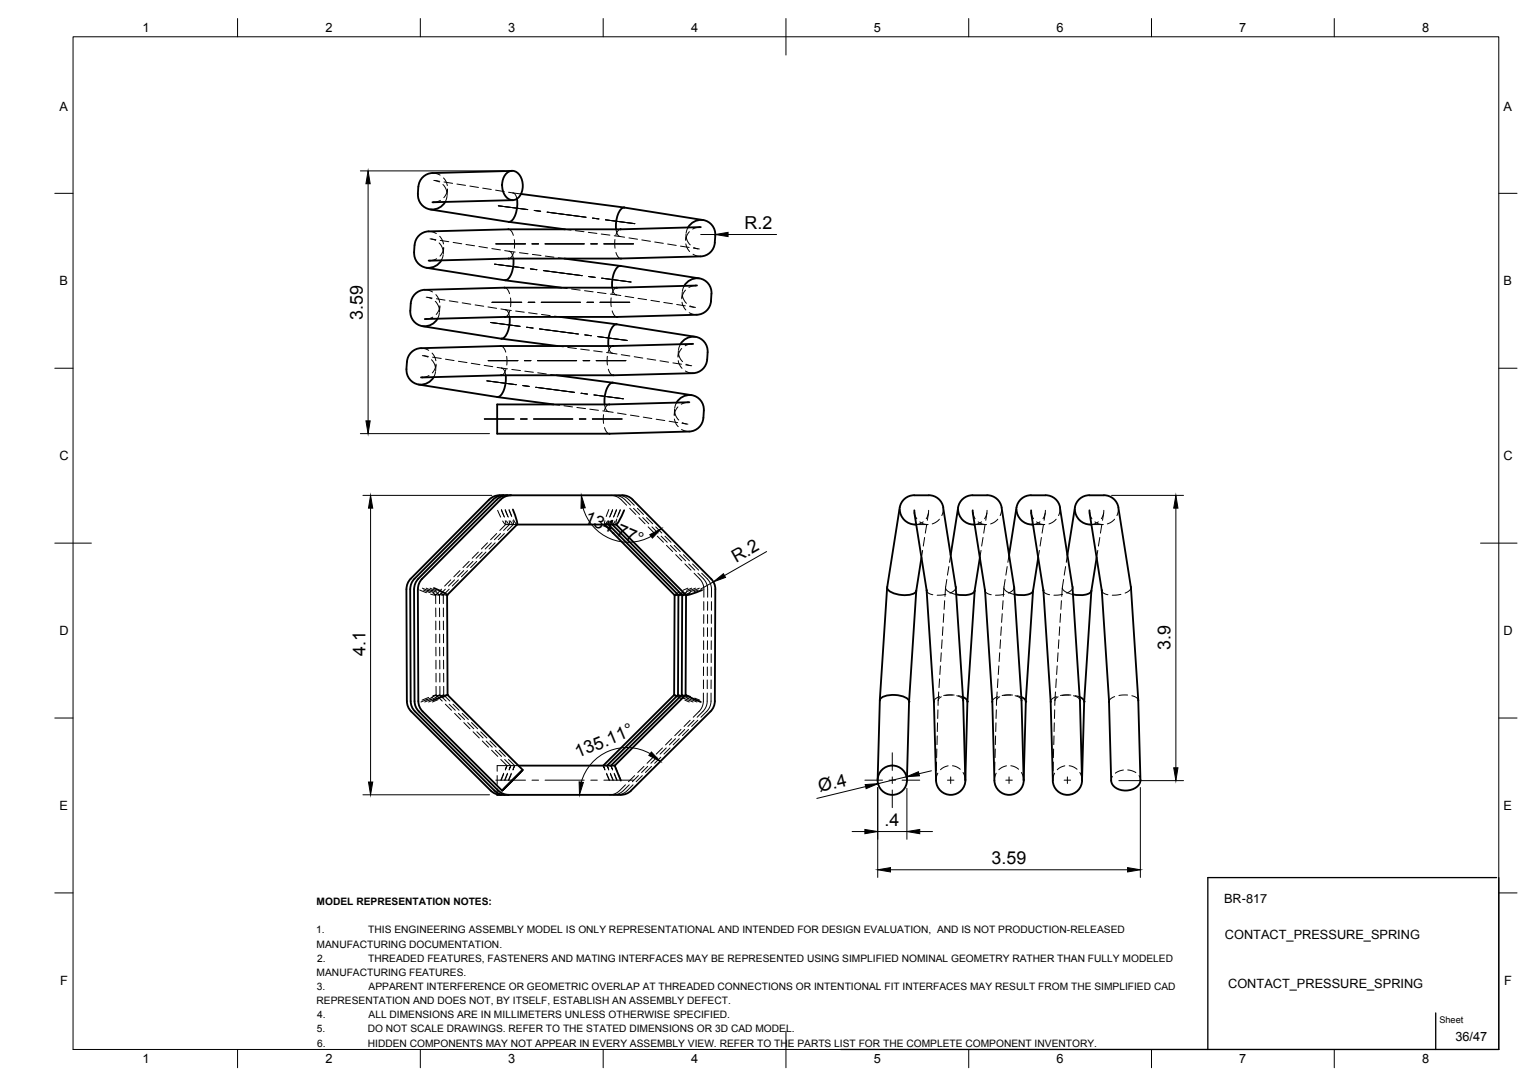
ISO-10303-21;
HEADER;
FILE_DESCRIPTION((''),'2;1');
FILE_NAME('CONTACT_PRESSURE_SPRING.step','2026-10-01T22:07:29-07:00',(''),(''),'','','');
FILE_SCHEMA (('AUTOMOTIVE_DESIGN { 1 0 10303 214 3 1 1 }'));
ENDSEC;
DATA;
#10=MECHANICAL_DESIGN_GEOMETRIC_PRESENTATION_REPRESENTATION('',(#569),#15484);
#131=ELLIPSE('',#9676,0.0216399563664951,0.02) ;
#132=ELLIPSE('',#9677,0.0216399563664951,0.02) ;
#133=ELLIPSE('',#9678,0.0216399563664951,0.02) ;
#134=ELLIPSE('',#9681,0.0216399563664949,0.02) ;
#135=ELLIPSE('',#9682,0.0216399563664949,0.02) ;
#136=ELLIPSE('',#9684,0.0216399563664949,0.02) ;
#137=ELLIPSE('',#9686,0.0216399563664949,0.02) ;
#138=ELLIPSE('',#9688,0.021639956366495,0.02) ;
#139=ELLIPSE('',#9690,0.021639956366495,0.02) ;
#140=ELLIPSE('',#9691,0.021639956366495,0.02) ;
#141=ELLIPSE('',#9693,0.0216399563664949,0.02) ;
#142=ELLIPSE('',#9694,0.0216399563664949,0.02) ;
#143=ELLIPSE('',#9695,0.0216399563664949,0.02) ;
#144=ELLIPSE('',#9697,0.021639956366495,0.02) ;
#145=ELLIPSE('',#9698,0.021639956366495,0.02) ;
#146=ELLIPSE('',#9700,0.0216399563664951,0.02) ;
#147=ELLIPSE('',#9701,0.0216399563664951,0.02) ;
#148=ELLIPSE('',#9702,0.0216399563664951,0.02) ;
#149=ELLIPSE('',#9704,0.0216399563664949,0.02) ;
#150=ELLIPSE('',#9705,0.0216399563664949,0.02) ;
#151=ELLIPSE('',#9707,0.0216399563664949,0.02) ;
#152=ELLIPSE('',#9709,0.021639956366495,0.02) ;
#153=ELLIPSE('',#9711,0.0216399563664949,0.02) ;
#154=ELLIPSE('',#9713,0.021639956366495,0.02) ;
#155=ELLIPSE('',#9714,0.021639956366495,0.02) ;
#156=ELLIPSE('',#9716,0.021639956366495,0.02) ;
#157=ELLIPSE('',#9717,0.021639956366495,0.02) ;
#158=ELLIPSE('',#9718,0.021639956366495,0.02) ;
#159=ELLIPSE('',#9720,0.021639956366495,0.02) ;
#160=ELLIPSE('',#9721,0.021639956366495,0.02) ;
#161=ELLIPSE('',#9723,0.021639956366495,0.02) ;
#162=ELLIPSE('',#9724,0.021639956366495,0.02) ;
#163=ELLIPSE('',#9725,0.021639956366495,0.02) ;
#164=ELLIPSE('',#9727,0.021639956366495,0.02) ;
#165=ELLIPSE('',#9728,0.021639956366495,0.02) ;
#166=ELLIPSE('',#9730,0.0216399563664949,0.02) ;
#167=ELLIPSE('',#9732,0.021639956366495,0.02) ;
#168=ELLIPSE('',#9734,0.0216399563664949,0.02) ;
#169=ELLIPSE('',#9736,0.021639956366495,0.02) ;
#170=ELLIPSE('',#9737,0.021639956366495,0.02) ;
#171=ELLIPSE('',#9739,0.0216399563664949,0.02) ;
#172=ELLIPSE('',#9740,0.0216399563664949,0.02) ;
#173=ELLIPSE('',#9741,0.0216399563664949,0.02) ;
#174=ELLIPSE('',#9743,0.0216399563664949,0.02) ;
#175=ELLIPSE('',#9744,0.0216399563664949,0.02) ;
#176=ELLIPSE('',#9746,0.0216399563664949,0.02) ;
#177=ELLIPSE('',#9747,0.0216399563664949,0.02) ;
#178=ELLIPSE('',#9748,0.0216399563664949,0.02) ;
#179=ELLIPSE('',#9750,0.021639956366495,0.02) ;
#180=ELLIPSE('',#9751,0.021639956366495,0.02) ;
#181=ELLIPSE('',#9753,0.0216399563664949,0.02) ;
#182=ELLIPSE('',#9755,0.0216399563664949,0.02) ;
#183=ELLIPSE('',#9757,0.0216399563664948,0.02) ;
#184=ELLIPSE('',#9759,0.021639956366495,0.02) ;
#185=ELLIPSE('',#9760,0.021639956366495,0.02) ;
#186=ELLIPSE('',#9762,0.0216399563664949,0.02) ;
#187=ELLIPSE('',#9763,0.0216399563664949,0.02) ;
#188=ELLIPSE('',#9764,0.0216399563664949,0.02) ;
#260=SPHERICAL_SURFACE('',#9549,0.02) ;
#261=SPHERICAL_SURFACE('',#9552,0.02) ;
#262=SPHERICAL_SURFACE('',#9556,0.02) ;
#263=SPHERICAL_SURFACE('',#9561,0.02) ;
#264=SPHERICAL_SURFACE('',#9566,0.02) ;
#265=SPHERICAL_SURFACE('',#9571,0.02) ;
#266=SPHERICAL_SURFACE('',#9575,0.02) ;
#267=SPHERICAL_SURFACE('',#9578,0.02) ;
#268=SPHERICAL_SURFACE('',#9581,0.02) ;
#269=SPHERICAL_SURFACE('',#9584,0.02) ;
#270=SPHERICAL_SURFACE('',#9588,0.02) ;
#271=SPHERICAL_SURFACE('',#9593,0.02) ;
#272=SPHERICAL_SURFACE('',#9598,0.02) ;
#273=SPHERICAL_SURFACE('',#9603,0.02) ;
#274=SPHERICAL_SURFACE('',#9607,0.02) ;
#275=SPHERICAL_SURFACE('',#9610,0.02) ;
#276=SPHERICAL_SURFACE('',#9613,0.02) ;
#277=SPHERICAL_SURFACE('',#9616,0.02) ;
#278=SPHERICAL_SURFACE('',#9620,0.02) ;
#279=SPHERICAL_SURFACE('',#9625,0.02) ;
#280=SPHERICAL_SURFACE('',#9630,0.02) ;
#281=SPHERICAL_SURFACE('',#9635,0.02) ;
#282=SPHERICAL_SURFACE('',#9639,0.02) ;
#283=SPHERICAL_SURFACE('',#9642,0.02) ;
#284=SPHERICAL_SURFACE('',#9645,0.02) ;
#285=SPHERICAL_SURFACE('',#9648,0.02) ;
#286=SPHERICAL_SURFACE('',#9652,0.02) ;
#287=SPHERICAL_SURFACE('',#9657,0.02) ;
#288=SPHERICAL_SURFACE('',#9662,0.02) ;
#289=SPHERICAL_SURFACE('',#9667,0.02) ;
#290=SPHERICAL_SURFACE('',#9671,0.02) ;
#498=SHAPE_REPRESENTATION_RELATIONSHIP('SRR','None',#15648,#533) ;
#533=ADVANCED_BREP_SHAPE_REPRESENTATION('',(#610),#15472) ;
#569=STYLED_ITEM('',(#15832),#610) ;
#610=MANIFOLD_SOLID_BREP('CONTACT_PRESSURE_SPRING',#8280) ;
#761=CYLINDRICAL_SURFACE('',#9674,0.02) ;
#762=CYLINDRICAL_SURFACE('',#9680,0.02) ;
#763=CYLINDRICAL_SURFACE('',#9683,0.02) ;
#764=CYLINDRICAL_SURFACE('',#9685,0.02) ;
#765=CYLINDRICAL_SURFACE('',#9687,0.02) ;
#766=CYLINDRICAL_SURFACE('',#9689,0.02) ;
#767=CYLINDRICAL_SURFACE('',#9692,0.02) ;
#768=CYLINDRICAL_SURFACE('',#9696,0.02) ;
#769=CYLINDRICAL_SURFACE('',#9699,0.02) ;
#770=CYLINDRICAL_SURFACE('',#9703,0.02) ;
#771=CYLINDRICAL_SURFACE('',#9706,0.02) ;
#772=CYLINDRICAL_SURFACE('',#9708,0.02) ;
#773=CYLINDRICAL_SURFACE('',#9710,0.02) ;
#774=CYLINDRICAL_SURFACE('',#9712,0.02) ;
#775=CYLINDRICAL_SURFACE('',#9715,0.02) ;
#776=CYLINDRICAL_SURFACE('',#9719,0.02) ;
#777=CYLINDRICAL_SURFACE('',#9722,0.02) ;
#778=CYLINDRICAL_SURFACE('',#9726,0.02) ;
#779=CYLINDRICAL_SURFACE('',#9729,0.02) ;
#780=CYLINDRICAL_SURFACE('',#9731,0.02) ;
#781=CYLINDRICAL_SURFACE('',#9733,0.02) ;
#782=CYLINDRICAL_SURFACE('',#9735,0.02) ;
#783=CYLINDRICAL_SURFACE('',#9738,0.02) ;
#784=CYLINDRICAL_SURFACE('',#9742,0.02) ;
#785=CYLINDRICAL_SURFACE('',#9745,0.02) ;
#786=CYLINDRICAL_SURFACE('',#9749,0.02) ;
#787=CYLINDRICAL_SURFACE('',#9752,0.02) ;
#788=CYLINDRICAL_SURFACE('',#9754,0.02) ;
#789=CYLINDRICAL_SURFACE('',#9756,0.02) ;
#790=CYLINDRICAL_SURFACE('',#9758,0.02) ;
#791=CYLINDRICAL_SURFACE('',#9761,0.02) ;
#792=CYLINDRICAL_SURFACE('',#9765,0.02) ;
#1229=CIRCLE('',#9550,0.02) ;
#1230=CIRCLE('',#9551,0.02) ;
#1231=CIRCLE('',#9553,0.02) ;
#1232=CIRCLE('',#9554,0.02) ;
#1233=CIRCLE('',#9555,0.02) ;
#1234=CIRCLE('',#9557,0.02) ;
#1235=CIRCLE('',#9558,0.02) ;
#1236=CIRCLE('',#9559,0.02) ;
#1237=CIRCLE('',#9560,0.02) ;
#1238=CIRCLE('',#9562,0.02) ;
#1239=CIRCLE('',#9563,0.02) ;
#1240=CIRCLE('',#9564,0.02) ;
#1241=CIRCLE('',#9565,0.02) ;
#1242=CIRCLE('',#9567,0.02) ;
#1243=CIRCLE('',#9568,0.02) ;
#1244=CIRCLE('',#9569,0.02) ;
#1245=CIRCLE('',#9570,0.02) ;
#1246=CIRCLE('',#9572,0.02) ;
#1247=CIRCLE('',#9573,0.02) ;
#1248=CIRCLE('',#9574,0.02) ;
#1249=CIRCLE('',#9576,0.02) ;
#1250=CIRCLE('',#9577,0.02) ;
#1251=CIRCLE('',#9579,0.02) ;
#1252=CIRCLE('',#9580,0.02) ;
#1253=CIRCLE('',#9582,0.02) ;
#1254=CIRCLE('',#9583,0.02) ;
#1255=CIRCLE('',#9585,0.02) ;
#1256=CIRCLE('',#9586,0.02) ;
#1257=CIRCLE('',#9587,0.02) ;
#1258=CIRCLE('',#9589,0.02) ;
#1259=CIRCLE('',#9590,0.02) ;
#1260=CIRCLE('',#9591,0.02) ;
#1261=CIRCLE('',#9592,0.02) ;
#1262=CIRCLE('',#9594,0.02) ;
#1263=CIRCLE('',#9595,0.02) ;
#1264=CIRCLE('',#9596,0.02) ;
#1265=CIRCLE('',#9597,0.02) ;
#1266=CIRCLE('',#9599,0.02) ;
#1267=CIRCLE('',#9600,0.02) ;
#1268=CIRCLE('',#9601,0.02) ;
#1269=CIRCLE('',#9602,0.02) ;
#1270=CIRCLE('',#9604,0.02) ;
#1271=CIRCLE('',#9605,0.02) ;
#1272=CIRCLE('',#9606,0.02) ;
#1273=CIRCLE('',#9608,0.02) ;
#1274=CIRCLE('',#9609,0.02) ;
#1275=CIRCLE('',#9611,0.02) ;
#1276=CIRCLE('',#9612,0.02) ;
#1277=CIRCLE('',#9614,0.02) ;
#1278=CIRCLE('',#9615,0.02) ;
#1279=CIRCLE('',#9617,0.02) ;
#1280=CIRCLE('',#9618,0.02) ;
#1281=CIRCLE('',#9619,0.02) ;
#1282=CIRCLE('',#9621,0.02) ;
#1283=CIRCLE('',#9622,0.02) ;
#1284=CIRCLE('',#9623,0.02) ;
#1285=CIRCLE('',#9624,0.02) ;
#1286=CIRCLE('',#9626,0.02) ;
#1287=CIRCLE('',#9627,0.02) ;
#1288=CIRCLE('',#9628,0.02) ;
#1289=CIRCLE('',#9629,0.02) ;
#1290=CIRCLE('',#9631,0.02) ;
#1291=CIRCLE('',#9632,0.02) ;
#1292=CIRCLE('',#9633,0.02) ;
#1293=CIRCLE('',#9634,0.02) ;
#1294=CIRCLE('',#9636,0.02) ;
#1295=CIRCLE('',#9637,0.02) ;
#1296=CIRCLE('',#9638,0.02) ;
#1297=CIRCLE('',#9640,0.02) ;
#1298=CIRCLE('',#9641,0.02) ;
#1299=CIRCLE('',#9643,0.02) ;
#1300=CIRCLE('',#9644,0.02) ;
#1301=CIRCLE('',#9646,0.02) ;
#1302=CIRCLE('',#9647,0.02) ;
#1303=CIRCLE('',#9649,0.02) ;
#1304=CIRCLE('',#9650,0.02) ;
#1305=CIRCLE('',#9651,0.02) ;
#1306=CIRCLE('',#9653,0.02) ;
#1307=CIRCLE('',#9654,0.02) ;
#1308=CIRCLE('',#9655,0.02) ;
#1309=CIRCLE('',#9656,0.02) ;
#1310=CIRCLE('',#9658,0.02) ;
#1311=CIRCLE('',#9659,0.02) ;
#1312=CIRCLE('',#9660,0.02) ;
#1313=CIRCLE('',#9661,0.02) ;
#1314=CIRCLE('',#9663,0.02) ;
#1315=CIRCLE('',#9664,0.02) ;
#1316=CIRCLE('',#9665,0.02) ;
#1317=CIRCLE('',#9666,0.02) ;
#1318=CIRCLE('',#9668,0.02) ;
#1319=CIRCLE('',#9669,0.02) ;
#1320=CIRCLE('',#9670,0.02) ;
#1321=CIRCLE('',#9672,0.02) ;
#1322=CIRCLE('',#9673,0.02) ;
#1323=CIRCLE('',#9675,0.02) ;
#1324=CIRCLE('',#9766,0.02) ;
#1724=FACE_OUTER_BOUND('',#2290,.T.) ;
#1725=FACE_OUTER_BOUND('',#2291,.T.) ;
#1726=FACE_OUTER_BOUND('',#2292,.T.) ;
#1727=FACE_OUTER_BOUND('',#2293,.T.) ;
#1728=FACE_OUTER_BOUND('',#2294,.T.) ;
#1729=FACE_OUTER_BOUND('',#2295,.T.) ;
#1730=FACE_OUTER_BOUND('',#2296,.T.) ;
#1731=FACE_OUTER_BOUND('',#2297,.T.) ;
#1732=FACE_OUTER_BOUND('',#2298,.T.) ;
#1733=FACE_OUTER_BOUND('',#2299,.T.) ;
#1734=FACE_OUTER_BOUND('',#2300,.T.) ;
#1735=FACE_OUTER_BOUND('',#2301,.T.) ;
#1736=FACE_OUTER_BOUND('',#2302,.T.) ;
#1737=FACE_OUTER_BOUND('',#2303,.T.) ;
#1738=FACE_OUTER_BOUND('',#2304,.T.) ;
#1739=FACE_OUTER_BOUND('',#2305,.T.) ;
#1740=FACE_OUTER_BOUND('',#2306,.T.) ;
#1741=FACE_OUTER_BOUND('',#2307,.T.) ;
#1742=FACE_OUTER_BOUND('',#2308,.T.) ;
#1743=FACE_OUTER_BOUND('',#2309,.T.) ;
#1744=FACE_OUTER_BOUND('',#2310,.T.) ;
#1745=FACE_OUTER_BOUND('',#2311,.T.) ;
#1746=FACE_OUTER_BOUND('',#2312,.T.) ;
#1747=FACE_OUTER_BOUND('',#2313,.T.) ;
#1748=FACE_OUTER_BOUND('',#2314,.T.) ;
#1749=FACE_OUTER_BOUND('',#2315,.T.) ;
#1750=FACE_OUTER_BOUND('',#2316,.T.) ;
#1751=FACE_OUTER_BOUND('',#2317,.T.) ;
#1752=FACE_OUTER_BOUND('',#2318,.T.) ;
#1753=FACE_OUTER_BOUND('',#2319,.T.) ;
#1754=FACE_OUTER_BOUND('',#2320,.T.) ;
#1755=FACE_OUTER_BOUND('',#2321,.T.) ;
#1756=FACE_OUTER_BOUND('',#2322,.T.) ;
#1757=FACE_OUTER_BOUND('',#2323,.T.) ;
#1758=FACE_OUTER_BOUND('',#2324,.T.) ;
#1759=FACE_OUTER_BOUND('',#2325,.T.) ;
#1760=FACE_OUTER_BOUND('',#2326,.T.) ;
#1761=FACE_OUTER_BOUND('',#2327,.T.) ;
#1762=FACE_OUTER_BOUND('',#2328,.T.) ;
#1763=FACE_OUTER_BOUND('',#2329,.T.) ;
#1764=FACE_OUTER_BOUND('',#2330,.T.) ;
#1765=FACE_OUTER_BOUND('',#2331,.T.) ;
#1766=FACE_OUTER_BOUND('',#2332,.T.) ;
#1767=FACE_OUTER_BOUND('',#2333,.T.) ;
#1768=FACE_OUTER_BOUND('',#2334,.T.) ;
#1769=FACE_OUTER_BOUND('',#2335,.T.) ;
#1770=FACE_OUTER_BOUND('',#2336,.T.) ;
#1771=FACE_OUTER_BOUND('',#2337,.T.) ;
#1772=FACE_OUTER_BOUND('',#2338,.T.) ;
#1773=FACE_OUTER_BOUND('',#2339,.T.) ;
#1774=FACE_OUTER_BOUND('',#2340,.T.) ;
#1775=FACE_OUTER_BOUND('',#2341,.T.) ;
#1776=FACE_OUTER_BOUND('',#2342,.T.) ;
#1777=FACE_OUTER_BOUND('',#2343,.T.) ;
#1778=FACE_OUTER_BOUND('',#2344,.T.) ;
#1779=FACE_OUTER_BOUND('',#2345,.T.) ;
#1780=FACE_OUTER_BOUND('',#2346,.T.) ;
#1781=FACE_OUTER_BOUND('',#2347,.T.) ;
#1782=FACE_OUTER_BOUND('',#2348,.T.) ;
#1783=FACE_OUTER_BOUND('',#2349,.T.) ;
#1784=FACE_OUTER_BOUND('',#2350,.T.) ;
#1785=FACE_OUTER_BOUND('',#2351,.T.) ;
#1786=FACE_OUTER_BOUND('',#2352,.T.) ;
#1787=FACE_OUTER_BOUND('',#2353,.T.) ;
#1788=FACE_OUTER_BOUND('',#2354,.T.) ;
#2290=EDGE_LOOP('',(#6897,#6898)) ;
#2291=EDGE_LOOP('',(#6899,#6900,#6901)) ;
#2292=EDGE_LOOP('',(#6902,#6903,#6904,#6905)) ;
#2293=EDGE_LOOP('',(#6906,#6907,#6908,#6909)) ;
#2294=EDGE_LOOP('',(#6910,#6911,#6912,#6913)) ;
#2295=EDGE_LOOP('',(#6914,#6915,#6916)) ;
#2296=EDGE_LOOP('',(#6917,#6918)) ;
#2297=EDGE_LOOP('',(#6919,#6920)) ;
#2298=EDGE_LOOP('',(#6921,#6922)) ;
#2299=EDGE_LOOP('',(#6923,#6924,#6925)) ;
#2300=EDGE_LOOP('',(#6926,#6927,#6928,#6929)) ;
#2301=EDGE_LOOP('',(#6930,#6931,#6932,#6933)) ;
#2302=EDGE_LOOP('',(#6934,#6935,#6936,#6937)) ;
#2303=EDGE_LOOP('',(#6938,#6939,#6940)) ;
#2304=EDGE_LOOP('',(#6941,#6942)) ;
#2305=EDGE_LOOP('',(#6943,#6944)) ;
#2306=EDGE_LOOP('',(#6945,#6946)) ;
#2307=EDGE_LOOP('',(#6947,#6948,#6949)) ;
#2308=EDGE_LOOP('',(#6950,#6951,#6952,#6953)) ;
#2309=EDGE_LOOP('',(#6954,#6955,#6956,#6957)) ;
#2310=EDGE_LOOP('',(#6958,#6959,#6960,#6961)) ;
#2311=EDGE_LOOP('',(#6962,#6963,#6964)) ;
#2312=EDGE_LOOP('',(#6965,#6966)) ;
#2313=EDGE_LOOP('',(#6967,#6968)) ;
#2314=EDGE_LOOP('',(#6969,#6970)) ;
#2315=EDGE_LOOP('',(#6971,#6972,#6973)) ;
#2316=EDGE_LOOP('',(#6974,#6975,#6976,#6977)) ;
#2317=EDGE_LOOP('',(#6978,#6979,#6980,#6981)) ;
#2318=EDGE_LOOP('',(#6982,#6983,#6984,#6985)) ;
#2319=EDGE_LOOP('',(#6986,#6987,#6988)) ;
#2320=EDGE_LOOP('',(#6989,#6990)) ;
#2321=EDGE_LOOP('',(#6991,#6992,#6993,#6994,#6995,#6996,#6997)) ;
#2322=EDGE_LOOP('',(#6998)) ;
#2323=EDGE_LOOP('',(#6999,#7000,#7001,#7002,#7003,#7004,#7005,#7006,#7007)) ;
#2324=EDGE_LOOP('',(#7008,#7009,#7010,#7011,#7012,#7013,#7014,#7015,#7016)) ;
#2325=EDGE_LOOP('',(#7017,#7018,#7019,#7020,#7021,#7022,#7023,#7024)) ;
#2326=EDGE_LOOP('',(#7025,#7026,#7027,#7028,#7029,#7030,#7031,#7032)) ;
#2327=EDGE_LOOP('',(#7033,#7034,#7035,#7036,#7037,#7038,#7039,#7040,#7041)) ;
#2328=EDGE_LOOP('',(#7042,#7043,#7044,#7045,#7046,#7047,#7048,#7049,#7050)) ;
#2329=EDGE_LOOP('',(#7051,#7052,#7053,#7054,#7055,#7056,#7057,#7058,#7059)) ;
#2330=EDGE_LOOP('',(#7060,#7061,#7062,#7063,#7064,#7065,#7066,#7067,#7068)) ;
#2331=EDGE_LOOP('',(#7069,#7070,#7071,#7072,#7073,#7074,#7075,#7076,#7077)) ;
#2332=EDGE_LOOP('',(#7078,#7079,#7080,#7081,#7082,#7083,#7084,#7085,#7086)) ;
#2333=EDGE_LOOP('',(#7087,#7088,#7089,#7090,#7091,#7092,#7093,#7094)) ;
#2334=EDGE_LOOP('',(#7095,#7096,#7097,#7098,#7099,#7100,#7101,#7102)) ;
#2335=EDGE_LOOP('',(#7103,#7104,#7105,#7106,#7107,#7108,#7109,#7110,#7111)) ;
#2336=EDGE_LOOP('',(#7112,#7113,#7114,#7115,#7116,#7117,#7118,#7119,#7120)) ;
#2337=EDGE_LOOP('',(#7121,#7122,#7123,#7124,#7125,#7126,#7127,#7128,#7129)) ;
#2338=EDGE_LOOP('',(#7130,#7131,#7132,#7133,#7134,#7135,#7136,#7137,#7138)) ;
#2339=EDGE_LOOP('',(#7139,#7140,#7141,#7142,#7143,#7144,#7145,#7146,#7147)) ;
#2340=EDGE_LOOP('',(#7148,#7149,#7150,#7151,#7152,#7153,#7154,#7155,#7156)) ;
#2341=EDGE_LOOP('',(#7157,#7158,#7159,#7160,#7161,#7162,#7163,#7164)) ;
#2342=EDGE_LOOP('',(#7165,#7166,#7167,#7168,#7169,#7170,#7171,#7172)) ;
#2343=EDGE_LOOP('',(#7173,#7174,#7175,#7176,#7177,#7178,#7179,#7180,#7181)) ;
#2344=EDGE_LOOP('',(#7182,#7183,#7184,#7185,#7186,#7187,#7188,#7189,#7190)) ;
#2345=EDGE_LOOP('',(#7191,#7192,#7193,#7194,#7195,#7196,#7197,#7198,#7199)) ;
#2346=EDGE_LOOP('',(#7200,#7201,#7202,#7203,#7204,#7205,#7206,#7207,#7208)) ;
#2347=EDGE_LOOP('',(#7209,#7210,#7211,#7212,#7213,#7214,#7215,#7216,#7217)) ;
#2348=EDGE_LOOP('',(#7218,#7219,#7220,#7221,#7222,#7223,#7224,#7225,#7226)) ;
#2349=EDGE_LOOP('',(#7227,#7228,#7229,#7230,#7231,#7232,#7233,#7234)) ;
#2350=EDGE_LOOP('',(#7235,#7236,#7237,#7238,#7239,#7240,#7241,#7242)) ;
#2351=EDGE_LOOP('',(#7243,#7244,#7245,#7246,#7247,#7248,#7249,#7250,#7251)) ;
#2352=EDGE_LOOP('',(#7252,#7253,#7254,#7255,#7256,#7257,#7258,#7259,#7260)) ;
#2353=EDGE_LOOP('',(#7261,#7262,#7263,#7264,#7265,#7266,#7267)) ;
#2354=EDGE_LOOP('',(#7268)) ;
#2788=LINE('',#14908,#3262) ;
#2789=LINE('',#14916,#3263) ;
#2790=LINE('',#14920,#3264) ;
#2791=LINE('',#14923,#3265) ;
#2792=LINE('',#14926,#3266) ;
#2793=LINE('',#14929,#3267) ;
#2794=LINE('',#14935,#3268) ;
#2795=LINE('',#14942,#3269) ;
#2796=LINE('',#14947,#3270) ;
#2797=LINE('',#14954,#3271) ;
#2798=LINE('',#14958,#3272) ;
#2799=LINE('',#14961,#3273) ;
#2800=LINE('',#14964,#3274) ;
#2801=LINE('',#14967,#3275) ;
#2802=LINE('',#14973,#3276) ;
#2803=LINE('',#14980,#3277) ;
#2804=LINE('',#14985,#3278) ;
#2805=LINE('',#14992,#3279) ;
#2806=LINE('',#14996,#3280) ;
#2807=LINE('',#14999,#3281) ;
#2808=LINE('',#15002,#3282) ;
#2809=LINE('',#15005,#3283) ;
#2810=LINE('',#15011,#3284) ;
#2811=LINE('',#15018,#3285) ;
#2812=LINE('',#15023,#3286) ;
#2813=LINE('',#15030,#3287) ;
#2814=LINE('',#15034,#3288) ;
#2815=LINE('',#15037,#3289) ;
#2816=LINE('',#15040,#3290) ;
#2817=LINE('',#15043,#3291) ;
#2818=LINE('',#15049,#3292) ;
#2819=LINE('',#15056,#3293) ;
#3262=VECTOR('',#12261,0.02) ;
#3263=VECTOR('',#12272,0.02) ;
#3264=VECTOR('',#12279,0.02) ;
#3265=VECTOR('',#12284,0.02) ;
#3266=VECTOR('',#12289,0.02) ;
#3267=VECTOR('',#12294,0.02) ;
#3268=VECTOR('',#12301,0.02) ;
#3269=VECTOR('',#12310,0.02) ;
#3270=VECTOR('',#12317,0.02) ;
#3271=VECTOR('',#12326,0.02) ;
#3272=VECTOR('',#12333,0.02) ;
#3273=VECTOR('',#12338,0.02) ;
#3274=VECTOR('',#12343,0.02) ;
#3275=VECTOR('',#12348,0.02) ;
#3276=VECTOR('',#12355,0.02) ;
#3277=VECTOR('',#12364,0.02) ;
#3278=VECTOR('',#12371,0.02) ;
#3279=VECTOR('',#12380,0.02) ;
#3280=VECTOR('',#12387,0.02) ;
#3281=VECTOR('',#12392,0.02) ;
#3282=VECTOR('',#12397,0.02) ;
#3283=VECTOR('',#12402,0.02) ;
#3284=VECTOR('',#12409,0.02) ;
#3285=VECTOR('',#12418,0.02) ;
#3286=VECTOR('',#12425,0.02) ;
#3287=VECTOR('',#12434,0.02) ;
#3288=VECTOR('',#12441,0.02) ;
#3289=VECTOR('',#12446,0.02) ;
#3290=VECTOR('',#12451,0.02) ;
#3291=VECTOR('',#12456,0.02) ;
#3292=VECTOR('',#12463,0.02) ;
#3293=VECTOR('',#12472,0.02) ;
#3929=VERTEX_POINT('',#14686) ;
#3930=VERTEX_POINT('',#14687) ;
#3931=VERTEX_POINT('',#14691) ;
#3932=VERTEX_POINT('',#14692) ;
#3933=VERTEX_POINT('',#14694) ;
#3934=VERTEX_POINT('',#14698) ;
#3935=VERTEX_POINT('',#14699) ;
#3936=VERTEX_POINT('',#14701) ;
#3937=VERTEX_POINT('',#14703) ;
#3938=VERTEX_POINT('',#14707) ;
#3939=VERTEX_POINT('',#14708) ;
#3940=VERTEX_POINT('',#14710) ;
#3941=VERTEX_POINT('',#14712) ;
#3942=VERTEX_POINT('',#14716) ;
#3943=VERTEX_POINT('',#14717) ;
#3944=VERTEX_POINT('',#14719) ;
#3945=VERTEX_POINT('',#14721) ;
#3946=VERTEX_POINT('',#14725) ;
#3947=VERTEX_POINT('',#14726) ;
#3948=VERTEX_POINT('',#14728) ;
#3949=VERTEX_POINT('',#14732) ;
#3950=VERTEX_POINT('',#14733) ;
#3951=VERTEX_POINT('',#14737) ;
#3952=VERTEX_POINT('',#14738) ;
#3953=VERTEX_POINT('',#14742) ;
#3954=VERTEX_POINT('',#14743) ;
#3955=VERTEX_POINT('',#14747) ;
#3956=VERTEX_POINT('',#14748) ;
#3957=VERTEX_POINT('',#14750) ;
#3958=VERTEX_POINT('',#14754) ;
#3959=VERTEX_POINT('',#14755) ;
#3960=VERTEX_POINT('',#14757) ;
#3961=VERTEX_POINT('',#14759) ;
#3962=VERTEX_POINT('',#14763) ;
#3963=VERTEX_POINT('',#14764) ;
#3964=VERTEX_POINT('',#14766) ;
#3965=VERTEX_POINT('',#14768) ;
#3966=VERTEX_POINT('',#14772) ;
#3967=VERTEX_POINT('',#14773) ;
#3968=VERTEX_POINT('',#14775) ;
#3969=VERTEX_POINT('',#14777) ;
#3970=VERTEX_POINT('',#14781) ;
#3971=VERTEX_POINT('',#14782) ;
#3972=VERTEX_POINT('',#14784) ;
#3973=VERTEX_POINT('',#14788) ;
#3974=VERTEX_POINT('',#14789) ;
#3975=VERTEX_POINT('',#14793) ;
#3976=VERTEX_POINT('',#14794) ;
#3977=VERTEX_POINT('',#14798) ;
#3978=VERTEX_POINT('',#14799) ;
#3979=VERTEX_POINT('',#14803) ;
#3980=VERTEX_POINT('',#14804) ;
#3981=VERTEX_POINT('',#14806) ;
#3982=VERTEX_POINT('',#14810) ;
#3983=VERTEX_POINT('',#14811) ;
#3984=VERTEX_POINT('',#14813) ;
#3985=VERTEX_POINT('',#14815) ;
#3986=VERTEX_POINT('',#14819) ;
#3987=VERTEX_POINT('',#14820) ;
#3988=VERTEX_POINT('',#14822) ;
#3989=VERTEX_POINT('',#14824) ;
#3990=VERTEX_POINT('',#14828) ;
#3991=VERTEX_POINT('',#14829) ;
#3992=VERTEX_POINT('',#14831) ;
#3993=VERTEX_POINT('',#14833) ;
#3994=VERTEX_POINT('',#14837) ;
#3995=VERTEX_POINT('',#14838) ;
#3996=VERTEX_POINT('',#14840) ;
#3997=VERTEX_POINT('',#14844) ;
#3998=VERTEX_POINT('',#14845) ;
#3999=VERTEX_POINT('',#14849) ;
#4000=VERTEX_POINT('',#14850) ;
#4001=VERTEX_POINT('',#14854) ;
#4002=VERTEX_POINT('',#14855) ;
#4003=VERTEX_POINT('',#14859) ;
#4004=VERTEX_POINT('',#14860) ;
#4005=VERTEX_POINT('',#14862) ;
#4006=VERTEX_POINT('',#14866) ;
#4007=VERTEX_POINT('',#14867) ;
#4008=VERTEX_POINT('',#14869) ;
#4009=VERTEX_POINT('',#14871) ;
#4010=VERTEX_POINT('',#14875) ;
#4011=VERTEX_POINT('',#14876) ;
#4012=VERTEX_POINT('',#14878) ;
#4013=VERTEX_POINT('',#14880) ;
#4014=VERTEX_POINT('',#14884) ;
#4015=VERTEX_POINT('',#14885) ;
#4016=VERTEX_POINT('',#14887) ;
#4017=VERTEX_POINT('',#14889) ;
#4018=VERTEX_POINT('',#14893) ;
#4019=VERTEX_POINT('',#14894) ;
#4020=VERTEX_POINT('',#14896) ;
#4021=VERTEX_POINT('',#14900) ;
#4022=VERTEX_POINT('',#14901) ;
#4023=VERTEX_POINT('',#14905) ;
#4024=VERTEX_POINT('',#14907) ;
#4025=VERTEX_POINT('',#14909) ;
#4026=VERTEX_POINT('',#14915) ;
#4027=VERTEX_POINT('',#14930) ;
#4028=VERTEX_POINT('',#14934) ;
#4029=VERTEX_POINT('',#14936) ;
#4030=VERTEX_POINT('',#14941) ;
#4031=VERTEX_POINT('',#14946) ;
#4032=VERTEX_POINT('',#14948) ;
#4033=VERTEX_POINT('',#14953) ;
#4034=VERTEX_POINT('',#14968) ;
#4035=VERTEX_POINT('',#14972) ;
#4036=VERTEX_POINT('',#14974) ;
#4037=VERTEX_POINT('',#14979) ;
#4038=VERTEX_POINT('',#14984) ;
#4039=VERTEX_POINT('',#14986) ;
#4040=VERTEX_POINT('',#14991) ;
#4041=VERTEX_POINT('',#15006) ;
#4042=VERTEX_POINT('',#15010) ;
#4043=VERTEX_POINT('',#15012) ;
#4044=VERTEX_POINT('',#15017) ;
#4045=VERTEX_POINT('',#15022) ;
#4046=VERTEX_POINT('',#15024) ;
#4047=VERTEX_POINT('',#15029) ;
#4048=VERTEX_POINT('',#15044) ;
#4049=VERTEX_POINT('',#15048) ;
#4050=VERTEX_POINT('',#15050) ;
#4051=VERTEX_POINT('',#15055) ;
#4953=EDGE_CURVE('',#3929,#3930,#1229,.T.) ;
#4954=EDGE_CURVE('',#3930,#3929,#1230,.T.) ;
#4955=EDGE_CURVE('',#3931,#3932,#1231,.T.) ;
#4956=EDGE_CURVE('',#3932,#3933,#1232,.T.) ;
#4957=EDGE_CURVE('',#3933,#3931,#1233,.T.) ;
#4958=EDGE_CURVE('',#3934,#3935,#1234,.T.) ;
#4959=EDGE_CURVE('',#3935,#3936,#1235,.T.) ;
#4960=EDGE_CURVE('',#3936,#3937,#1236,.T.) ;
#4961=EDGE_CURVE('',#3937,#3934,#1237,.T.) ;
#4962=EDGE_CURVE('',#3938,#3939,#1238,.T.) ;
#4963=EDGE_CURVE('',#3939,#3940,#1239,.T.) ;
#4964=EDGE_CURVE('',#3940,#3941,#1240,.T.) ;
#4965=EDGE_CURVE('',#3941,#3938,#1241,.T.) ;
#4966=EDGE_CURVE('',#3942,#3943,#1242,.T.) ;
#4967=EDGE_CURVE('',#3943,#3944,#1243,.T.) ;
#4968=EDGE_CURVE('',#3944,#3945,#1244,.T.) ;
#4969=EDGE_CURVE('',#3945,#3942,#1245,.T.) ;
#4970=EDGE_CURVE('',#3946,#3947,#1246,.T.) ;
#4971=EDGE_CURVE('',#3947,#3948,#1247,.T.) ;
#4972=EDGE_CURVE('',#3948,#3946,#1248,.T.) ;
#4973=EDGE_CURVE('',#3949,#3950,#1249,.T.) ;
#4974=EDGE_CURVE('',#3950,#3949,#1250,.T.) ;
#4975=EDGE_CURVE('',#3951,#3952,#1251,.T.) ;
#4976=EDGE_CURVE('',#3952,#3951,#1252,.T.) ;
#4977=EDGE_CURVE('',#3953,#3954,#1253,.T.) ;
#4978=EDGE_CURVE('',#3954,#3953,#1254,.T.) ;
#4979=EDGE_CURVE('',#3955,#3956,#1255,.T.) ;
#4980=EDGE_CURVE('',#3956,#3957,#1256,.T.) ;
#4981=EDGE_CURVE('',#3957,#3955,#1257,.T.) ;
#4982=EDGE_CURVE('',#3958,#3959,#1258,.T.) ;
#4983=EDGE_CURVE('',#3959,#3960,#1259,.T.) ;
#4984=EDGE_CURVE('',#3960,#3961,#1260,.T.) ;
#4985=EDGE_CURVE('',#3961,#3958,#1261,.T.) ;
#4986=EDGE_CURVE('',#3962,#3963,#1262,.T.) ;
#4987=EDGE_CURVE('',#3963,#3964,#1263,.T.) ;
#4988=EDGE_CURVE('',#3964,#3965,#1264,.T.) ;
#4989=EDGE_CURVE('',#3965,#3962,#1265,.T.) ;
#4990=EDGE_CURVE('',#3966,#3967,#1266,.T.) ;
#4991=EDGE_CURVE('',#3967,#3968,#1267,.T.) ;
#4992=EDGE_CURVE('',#3968,#3969,#1268,.T.) ;
#4993=EDGE_CURVE('',#3969,#3966,#1269,.T.) ;
#4994=EDGE_CURVE('',#3970,#3971,#1270,.T.) ;
#4995=EDGE_CURVE('',#3971,#3972,#1271,.T.) ;
#4996=EDGE_CURVE('',#3972,#3970,#1272,.T.) ;
#4997=EDGE_CURVE('',#3973,#3974,#1273,.T.) ;
#4998=EDGE_CURVE('',#3974,#3973,#1274,.T.) ;
#4999=EDGE_CURVE('',#3975,#3976,#1275,.T.) ;
#5000=EDGE_CURVE('',#3976,#3975,#1276,.T.) ;
#5001=EDGE_CURVE('',#3977,#3978,#1277,.T.) ;
#5002=EDGE_CURVE('',#3978,#3977,#1278,.T.) ;
#5003=EDGE_CURVE('',#3979,#3980,#1279,.T.) ;
#5004=EDGE_CURVE('',#3980,#3981,#1280,.T.) ;
#5005=EDGE_CURVE('',#3981,#3979,#1281,.T.) ;
#5006=EDGE_CURVE('',#3982,#3983,#1282,.T.) ;
#5007=EDGE_CURVE('',#3983,#3984,#1283,.T.) ;
#5008=EDGE_CURVE('',#3984,#3985,#1284,.T.) ;
#5009=EDGE_CURVE('',#3985,#3982,#1285,.T.) ;
#5010=EDGE_CURVE('',#3986,#3987,#1286,.T.) ;
#5011=EDGE_CURVE('',#3987,#3988,#1287,.T.) ;
#5012=EDGE_CURVE('',#3988,#3989,#1288,.T.) ;
#5013=EDGE_CURVE('',#3989,#3986,#1289,.T.) ;
#5014=EDGE_CURVE('',#3990,#3991,#1290,.T.) ;
#5015=EDGE_CURVE('',#3991,#3992,#1291,.T.) ;
#5016=EDGE_CURVE('',#3992,#3993,#1292,.T.) ;
#5017=EDGE_CURVE('',#3993,#3990,#1293,.T.) ;
#5018=EDGE_CURVE('',#3994,#3995,#1294,.T.) ;
#5019=EDGE_CURVE('',#3995,#3996,#1295,.T.) ;
#5020=EDGE_CURVE('',#3996,#3994,#1296,.T.) ;
#5021=EDGE_CURVE('',#3997,#3998,#1297,.T.) ;
#5022=EDGE_CURVE('',#3998,#3997,#1298,.T.) ;
#5023=EDGE_CURVE('',#3999,#4000,#1299,.T.) ;
#5024=EDGE_CURVE('',#4000,#3999,#1300,.T.) ;
#5025=EDGE_CURVE('',#4001,#4002,#1301,.T.) ;
#5026=EDGE_CURVE('',#4002,#4001,#1302,.T.) ;
#5027=EDGE_CURVE('',#4003,#4004,#1303,.T.) ;
#5028=EDGE_CURVE('',#4004,#4005,#1304,.T.) ;
#5029=EDGE_CURVE('',#4005,#4003,#1305,.T.) ;
#5030=EDGE_CURVE('',#4006,#4007,#1306,.T.) ;
#5031=EDGE_CURVE('',#4007,#4008,#1307,.T.) ;
#5032=EDGE_CURVE('',#4008,#4009,#1308,.T.) ;
#5033=EDGE_CURVE('',#4009,#4006,#1309,.T.) ;
#5034=EDGE_CURVE('',#4010,#4011,#1310,.T.) ;
#5035=EDGE_CURVE('',#4011,#4012,#1311,.T.) ;
#5036=EDGE_CURVE('',#4012,#4013,#1312,.T.) ;
#5037=EDGE_CURVE('',#4013,#4010,#1313,.T.) ;
#5038=EDGE_CURVE('',#4014,#4015,#1314,.T.) ;
#5039=EDGE_CURVE('',#4015,#4016,#1315,.T.) ;
#5040=EDGE_CURVE('',#4016,#4017,#1316,.T.) ;
#5041=EDGE_CURVE('',#4017,#4014,#1317,.T.) ;
#5042=EDGE_CURVE('',#4018,#4019,#1318,.T.) ;
#5043=EDGE_CURVE('',#4019,#4020,#1319,.T.) ;
#5044=EDGE_CURVE('',#4020,#4018,#1320,.T.) ;
#5045=EDGE_CURVE('',#4021,#4022,#1321,.T.) ;
#5046=EDGE_CURVE('',#4022,#4021,#1322,.T.) ;
#5047=EDGE_CURVE('',#4023,#4023,#1323,.T.) ;
#5048=EDGE_CURVE('',#4023,#4024,#2788,.T.) ;
#5049=EDGE_CURVE('',#4025,#4024,#131,.T.) ;
#5050=EDGE_CURVE('',#3930,#4025,#132,.T.) ;
#5051=EDGE_CURVE('',#4024,#3929,#133,.T.) ;
#5052=EDGE_CURVE('',#4025,#4026,#2789,.T.) ;
#5053=EDGE_CURVE('',#3932,#4026,#134,.T.) ;
#5054=EDGE_CURVE('',#4026,#3931,#135,.T.) ;
#5055=EDGE_CURVE('',#3933,#3935,#2790,.T.) ;
#5056=EDGE_CURVE('',#3936,#3934,#136,.T.) ;
#5057=EDGE_CURVE('',#3937,#3939,#2791,.T.) ;
#5058=EDGE_CURVE('',#3940,#3938,#137,.T.) ;
#5059=EDGE_CURVE('',#3941,#3943,#2792,.T.) ;
#5060=EDGE_CURVE('',#3944,#3942,#138,.T.) ;
#5061=EDGE_CURVE('',#3945,#3947,#2793,.T.) ;
#5062=EDGE_CURVE('',#4027,#3946,#139,.T.) ;
#5063=EDGE_CURVE('',#3948,#4027,#140,.T.) ;
#5064=EDGE_CURVE('',#4027,#4028,#2794,.T.) ;
#5065=EDGE_CURVE('',#4029,#4028,#141,.T.) ;
#5066=EDGE_CURVE('',#3950,#4029,#142,.T.) ;
#5067=EDGE_CURVE('',#4028,#3949,#143,.T.) ;
#5068=EDGE_CURVE('',#4029,#4030,#2795,.T.) ;
#5069=EDGE_CURVE('',#3952,#4030,#144,.T.) ;
#5070=EDGE_CURVE('',#4030,#3951,#145,.T.) ;
#5071=EDGE_CURVE('',#4030,#4031,#2796,.T.) ;
#5072=EDGE_CURVE('',#4032,#4031,#146,.T.) ;
#5073=EDGE_CURVE('',#3954,#4032,#147,.T.) ;
#5074=EDGE_CURVE('',#4031,#3953,#148,.T.) ;
#5075=EDGE_CURVE('',#4032,#4033,#2797,.T.) ;
#5076=EDGE_CURVE('',#3956,#4033,#149,.T.) ;
#5077=EDGE_CURVE('',#4033,#3955,#150,.T.) ;
#5078=EDGE_CURVE('',#3957,#3959,#2798,.T.) ;
#5079=EDGE_CURVE('',#3960,#3958,#151,.T.) ;
#5080=EDGE_CURVE('',#3961,#3963,#2799,.T.) ;
#5081=EDGE_CURVE('',#3964,#3962,#152,.T.) ;
#5082=EDGE_CURVE('',#3965,#3967,#2800,.T.) ;
#5083=EDGE_CURVE('',#3968,#3966,#153,.T.) ;
#5084=EDGE_CURVE('',#3969,#3971,#2801,.T.) ;
#5085=EDGE_CURVE('',#4034,#3970,#154,.T.) ;
#5086=EDGE_CURVE('',#3972,#4034,#155,.T.) ;
#5087=EDGE_CURVE('',#4034,#4035,#2802,.T.) ;
#5088=EDGE_CURVE('',#4036,#4035,#156,.T.) ;
#5089=EDGE_CURVE('',#3974,#4036,#157,.T.) ;
#5090=EDGE_CURVE('',#4035,#3973,#158,.T.) ;
#5091=EDGE_CURVE('',#4036,#4037,#2803,.T.) ;
#5092=EDGE_CURVE('',#3976,#4037,#159,.T.) ;
#5093=EDGE_CURVE('',#4037,#3975,#160,.T.) ;
#5094=EDGE_CURVE('',#4037,#4038,#2804,.T.) ;
#5095=EDGE_CURVE('',#4039,#4038,#161,.T.) ;
#5096=EDGE_CURVE('',#3978,#4039,#162,.T.) ;
#5097=EDGE_CURVE('',#4038,#3977,#163,.T.) ;
#5098=EDGE_CURVE('',#4039,#4040,#2805,.T.) ;
#5099=EDGE_CURVE('',#3980,#4040,#164,.T.) ;
#5100=EDGE_CURVE('',#4040,#3979,#165,.T.) ;
#5101=EDGE_CURVE('',#3981,#3983,#2806,.T.) ;
#5102=EDGE_CURVE('',#3984,#3982,#166,.T.) ;
#5103=EDGE_CURVE('',#3985,#3987,#2807,.T.) ;
#5104=EDGE_CURVE('',#3988,#3986,#167,.T.) ;
#5105=EDGE_CURVE('',#3989,#3991,#2808,.T.) ;
#5106=EDGE_CURVE('',#3992,#3990,#168,.T.) ;
#5107=EDGE_CURVE('',#3993,#3995,#2809,.T.) ;
#5108=EDGE_CURVE('',#4041,#3994,#169,.T.) ;
#5109=EDGE_CURVE('',#3996,#4041,#170,.T.) ;
#5110=EDGE_CURVE('',#4041,#4042,#2810,.T.) ;
#5111=EDGE_CURVE('',#4043,#4042,#171,.T.) ;
#5112=EDGE_CURVE('',#3998,#4043,#172,.T.) ;
#5113=EDGE_CURVE('',#4042,#3997,#173,.T.) ;
#5114=EDGE_CURVE('',#4043,#4044,#2811,.T.) ;
#5115=EDGE_CURVE('',#4000,#4044,#174,.T.) ;
#5116=EDGE_CURVE('',#4044,#3999,#175,.T.) ;
#5117=EDGE_CURVE('',#4044,#4045,#2812,.T.) ;
#5118=EDGE_CURVE('',#4046,#4045,#176,.T.) ;
#5119=EDGE_CURVE('',#4002,#4046,#177,.T.) ;
#5120=EDGE_CURVE('',#4045,#4001,#178,.T.) ;
#5121=EDGE_CURVE('',#4046,#4047,#2813,.T.) ;
#5122=EDGE_CURVE('',#4004,#4047,#179,.T.) ;
#5123=EDGE_CURVE('',#4047,#4003,#180,.T.) ;
#5124=EDGE_CURVE('',#4005,#4007,#2814,.T.) ;
#5125=EDGE_CURVE('',#4008,#4006,#181,.T.) ;
#5126=EDGE_CURVE('',#4009,#4011,#2815,.T.) ;
#5127=EDGE_CURVE('',#4012,#4010,#182,.T.) ;
#5128=EDGE_CURVE('',#4013,#4015,#2816,.T.) ;
#5129=EDGE_CURVE('',#4016,#4014,#183,.T.) ;
#5130=EDGE_CURVE('',#4017,#4019,#2817,.T.) ;
#5131=EDGE_CURVE('',#4048,#4018,#184,.T.) ;
#5132=EDGE_CURVE('',#4020,#4048,#185,.T.) ;
#5133=EDGE_CURVE('',#4048,#4049,#2818,.T.) ;
#5134=EDGE_CURVE('',#4050,#4049,#186,.T.) ;
#5135=EDGE_CURVE('',#4022,#4050,#187,.T.) ;
#5136=EDGE_CURVE('',#4049,#4021,#188,.T.) ;
#5137=EDGE_CURVE('',#4050,#4051,#2819,.T.) ;
#5138=EDGE_CURVE('',#4051,#4051,#1324,.T.) ;
#6897=ORIENTED_EDGE('',*,*,#4953,.T.) ;
#6898=ORIENTED_EDGE('',*,*,#4954,.T.) ;
#6899=ORIENTED_EDGE('',*,*,#4955,.T.) ;
#6900=ORIENTED_EDGE('',*,*,#4956,.T.) ;
#6901=ORIENTED_EDGE('',*,*,#4957,.T.) ;
#6902=ORIENTED_EDGE('',*,*,#4958,.T.) ;
#6903=ORIENTED_EDGE('',*,*,#4959,.T.) ;
#6904=ORIENTED_EDGE('',*,*,#4960,.T.) ;
#6905=ORIENTED_EDGE('',*,*,#4961,.T.) ;
#6906=ORIENTED_EDGE('',*,*,#4962,.T.) ;
#6907=ORIENTED_EDGE('',*,*,#4963,.T.) ;
#6908=ORIENTED_EDGE('',*,*,#4964,.T.) ;
#6909=ORIENTED_EDGE('',*,*,#4965,.T.) ;
#6910=ORIENTED_EDGE('',*,*,#4966,.T.) ;
#6911=ORIENTED_EDGE('',*,*,#4967,.T.) ;
#6912=ORIENTED_EDGE('',*,*,#4968,.T.) ;
#6913=ORIENTED_EDGE('',*,*,#4969,.T.) ;
#6914=ORIENTED_EDGE('',*,*,#4970,.T.) ;
#6915=ORIENTED_EDGE('',*,*,#4971,.T.) ;
#6916=ORIENTED_EDGE('',*,*,#4972,.T.) ;
#6917=ORIENTED_EDGE('',*,*,#4973,.T.) ;
#6918=ORIENTED_EDGE('',*,*,#4974,.T.) ;
#6919=ORIENTED_EDGE('',*,*,#4975,.T.) ;
#6920=ORIENTED_EDGE('',*,*,#4976,.T.) ;
#6921=ORIENTED_EDGE('',*,*,#4977,.T.) ;
#6922=ORIENTED_EDGE('',*,*,#4978,.T.) ;
#6923=ORIENTED_EDGE('',*,*,#4979,.T.) ;
#6924=ORIENTED_EDGE('',*,*,#4980,.T.) ;
#6925=ORIENTED_EDGE('',*,*,#4981,.T.) ;
#6926=ORIENTED_EDGE('',*,*,#4982,.T.) ;
#6927=ORIENTED_EDGE('',*,*,#4983,.T.) ;
#6928=ORIENTED_EDGE('',*,*,#4984,.T.) ;
#6929=ORIENTED_EDGE('',*,*,#4985,.T.) ;
#6930=ORIENTED_EDGE('',*,*,#4986,.T.) ;
#6931=ORIENTED_EDGE('',*,*,#4987,.T.) ;
#6932=ORIENTED_EDGE('',*,*,#4988,.T.) ;
#6933=ORIENTED_EDGE('',*,*,#4989,.T.) ;
#6934=ORIENTED_EDGE('',*,*,#4990,.T.) ;
#6935=ORIENTED_EDGE('',*,*,#4991,.T.) ;
#6936=ORIENTED_EDGE('',*,*,#4992,.T.) ;
#6937=ORIENTED_EDGE('',*,*,#4993,.T.) ;
#6938=ORIENTED_EDGE('',*,*,#4994,.T.) ;
#6939=ORIENTED_EDGE('',*,*,#4995,.T.) ;
#6940=ORIENTED_EDGE('',*,*,#4996,.T.) ;
#6941=ORIENTED_EDGE('',*,*,#4997,.T.) ;
#6942=ORIENTED_EDGE('',*,*,#4998,.T.) ;
#6943=ORIENTED_EDGE('',*,*,#4999,.T.) ;
#6944=ORIENTED_EDGE('',*,*,#5000,.T.) ;
#6945=ORIENTED_EDGE('',*,*,#5001,.T.) ;
#6946=ORIENTED_EDGE('',*,*,#5002,.T.) ;
#6947=ORIENTED_EDGE('',*,*,#5003,.T.) ;
#6948=ORIENTED_EDGE('',*,*,#5004,.T.) ;
#6949=ORIENTED_EDGE('',*,*,#5005,.T.) ;
#6950=ORIENTED_EDGE('',*,*,#5006,.T.) ;
#6951=ORIENTED_EDGE('',*,*,#5007,.T.) ;
#6952=ORIENTED_EDGE('',*,*,#5008,.T.) ;
#6953=ORIENTED_EDGE('',*,*,#5009,.T.) ;
#6954=ORIENTED_EDGE('',*,*,#5010,.T.) ;
#6955=ORIENTED_EDGE('',*,*,#5011,.T.) ;
#6956=ORIENTED_EDGE('',*,*,#5012,.T.) ;
#6957=ORIENTED_EDGE('',*,*,#5013,.T.) ;
#6958=ORIENTED_EDGE('',*,*,#5014,.T.) ;
#6959=ORIENTED_EDGE('',*,*,#5015,.T.) ;
#6960=ORIENTED_EDGE('',*,*,#5016,.T.) ;
#6961=ORIENTED_EDGE('',*,*,#5017,.T.) ;
#6962=ORIENTED_EDGE('',*,*,#5018,.T.) ;
#6963=ORIENTED_EDGE('',*,*,#5019,.T.) ;
#6964=ORIENTED_EDGE('',*,*,#5020,.T.) ;
#6965=ORIENTED_EDGE('',*,*,#5021,.T.) ;
#6966=ORIENTED_EDGE('',*,*,#5022,.T.) ;
#6967=ORIENTED_EDGE('',*,*,#5023,.T.) ;
#6968=ORIENTED_EDGE('',*,*,#5024,.T.) ;
#6969=ORIENTED_EDGE('',*,*,#5025,.T.) ;
#6970=ORIENTED_EDGE('',*,*,#5026,.T.) ;
#6971=ORIENTED_EDGE('',*,*,#5027,.T.) ;
#6972=ORIENTED_EDGE('',*,*,#5028,.T.) ;
#6973=ORIENTED_EDGE('',*,*,#5029,.T.) ;
#6974=ORIENTED_EDGE('',*,*,#5030,.T.) ;
#6975=ORIENTED_EDGE('',*,*,#5031,.T.) ;
#6976=ORIENTED_EDGE('',*,*,#5032,.T.) ;
#6977=ORIENTED_EDGE('',*,*,#5033,.T.) ;
#6978=ORIENTED_EDGE('',*,*,#5034,.T.) ;
#6979=ORIENTED_EDGE('',*,*,#5035,.T.) ;
#6980=ORIENTED_EDGE('',*,*,#5036,.T.) ;
#6981=ORIENTED_EDGE('',*,*,#5037,.T.) ;
#6982=ORIENTED_EDGE('',*,*,#5038,.T.) ;
#6983=ORIENTED_EDGE('',*,*,#5039,.T.) ;
#6984=ORIENTED_EDGE('',*,*,#5040,.T.) ;
#6985=ORIENTED_EDGE('',*,*,#5041,.T.) ;
#6986=ORIENTED_EDGE('',*,*,#5042,.T.) ;
#6987=ORIENTED_EDGE('',*,*,#5043,.T.) ;
#6988=ORIENTED_EDGE('',*,*,#5044,.T.) ;
#6989=ORIENTED_EDGE('',*,*,#5045,.T.) ;
#6990=ORIENTED_EDGE('',*,*,#5046,.T.) ;
#6991=ORIENTED_EDGE('',*,*,#5047,.F.) ;
#6992=ORIENTED_EDGE('',*,*,#5048,.T.) ;
#6993=ORIENTED_EDGE('',*,*,#5049,.F.) ;
#6994=ORIENTED_EDGE('',*,*,#5050,.F.) ;
#6995=ORIENTED_EDGE('',*,*,#4953,.F.) ;
#6996=ORIENTED_EDGE('',*,*,#5051,.F.) ;
#6997=ORIENTED_EDGE('',*,*,#5048,.F.) ;
#6998=ORIENTED_EDGE('',*,*,#5047,.T.) ;
#6999=ORIENTED_EDGE('',*,*,#5050,.T.) ;
#7000=ORIENTED_EDGE('',*,*,#5052,.T.) ;
#7001=ORIENTED_EDGE('',*,*,#5053,.F.) ;
#7002=ORIENTED_EDGE('',*,*,#4955,.F.) ;
#7003=ORIENTED_EDGE('',*,*,#5054,.F.) ;
#7004=ORIENTED_EDGE('',*,*,#5052,.F.) ;
#7005=ORIENTED_EDGE('',*,*,#5049,.T.) ;
#7006=ORIENTED_EDGE('',*,*,#5051,.T.) ;
#7007=ORIENTED_EDGE('',*,*,#4954,.F.) ;
#7008=ORIENTED_EDGE('',*,*,#5053,.T.) ;
#7009=ORIENTED_EDGE('',*,*,#5054,.T.) ;
#7010=ORIENTED_EDGE('',*,*,#4957,.F.) ;
#7011=ORIENTED_EDGE('',*,*,#5055,.T.) ;
#7012=ORIENTED_EDGE('',*,*,#4958,.F.) ;
#7013=ORIENTED_EDGE('',*,*,#5056,.F.) ;
#7014=ORIENTED_EDGE('',*,*,#4959,.F.) ;
#7015=ORIENTED_EDGE('',*,*,#5055,.F.) ;
#7016=ORIENTED_EDGE('',*,*,#4956,.F.) ;
#7017=ORIENTED_EDGE('',*,*,#5056,.T.) ;
#7018=ORIENTED_EDGE('',*,*,#4961,.F.) ;
#7019=ORIENTED_EDGE('',*,*,#5057,.T.) ;
#7020=ORIENTED_EDGE('',*,*,#4962,.F.) ;
#7021=ORIENTED_EDGE('',*,*,#5058,.F.) ;
#7022=ORIENTED_EDGE('',*,*,#4963,.F.) ;
#7023=ORIENTED_EDGE('',*,*,#5057,.F.) ;
#7024=ORIENTED_EDGE('',*,*,#4960,.F.) ;
#7025=ORIENTED_EDGE('',*,*,#5058,.T.) ;
#7026=ORIENTED_EDGE('',*,*,#4965,.F.) ;
#7027=ORIENTED_EDGE('',*,*,#5059,.T.) ;
#7028=ORIENTED_EDGE('',*,*,#4966,.F.) ;
#7029=ORIENTED_EDGE('',*,*,#5060,.F.) ;
#7030=ORIENTED_EDGE('',*,*,#4967,.F.) ;
#7031=ORIENTED_EDGE('',*,*,#5059,.F.) ;
#7032=ORIENTED_EDGE('',*,*,#4964,.F.) ;
#7033=ORIENTED_EDGE('',*,*,#5060,.T.) ;
#7034=ORIENTED_EDGE('',*,*,#4969,.F.) ;
#7035=ORIENTED_EDGE('',*,*,#5061,.T.) ;
#7036=ORIENTED_EDGE('',*,*,#4970,.F.) ;
#7037=ORIENTED_EDGE('',*,*,#5062,.F.) ;
#7038=ORIENTED_EDGE('',*,*,#5063,.F.) ;
#7039=ORIENTED_EDGE('',*,*,#4971,.F.) ;
#7040=ORIENTED_EDGE('',*,*,#5061,.F.) ;
#7041=ORIENTED_EDGE('',*,*,#4968,.F.) ;
#7042=ORIENTED_EDGE('',*,*,#5063,.T.) ;
#7043=ORIENTED_EDGE('',*,*,#5064,.T.) ;
#7044=ORIENTED_EDGE('',*,*,#5065,.F.) ;
#7045=ORIENTED_EDGE('',*,*,#5066,.F.) ;
#7046=ORIENTED_EDGE('',*,*,#4973,.F.) ;
#7047=ORIENTED_EDGE('',*,*,#5067,.F.) ;
#7048=ORIENTED_EDGE('',*,*,#5064,.F.) ;
#7049=ORIENTED_EDGE('',*,*,#5062,.T.) ;
#7050=ORIENTED_EDGE('',*,*,#4972,.F.) ;
#7051=ORIENTED_EDGE('',*,*,#5066,.T.) ;
#7052=ORIENTED_EDGE('',*,*,#5068,.T.) ;
#7053=ORIENTED_EDGE('',*,*,#5069,.F.) ;
#7054=ORIENTED_EDGE('',*,*,#4975,.F.) ;
#7055=ORIENTED_EDGE('',*,*,#5070,.F.) ;
#7056=ORIENTED_EDGE('',*,*,#5068,.F.) ;
#7057=ORIENTED_EDGE('',*,*,#5065,.T.) ;
#7058=ORIENTED_EDGE('',*,*,#5067,.T.) ;
#7059=ORIENTED_EDGE('',*,*,#4974,.F.) ;
#7060=ORIENTED_EDGE('',*,*,#5069,.T.) ;
#7061=ORIENTED_EDGE('',*,*,#5071,.T.) ;
#7062=ORIENTED_EDGE('',*,*,#5072,.F.) ;
#7063=ORIENTED_EDGE('',*,*,#5073,.F.) ;
#7064=ORIENTED_EDGE('',*,*,#4977,.F.) ;
#7065=ORIENTED_EDGE('',*,*,#5074,.F.) ;
#7066=ORIENTED_EDGE('',*,*,#5071,.F.) ;
#7067=ORIENTED_EDGE('',*,*,#5070,.T.) ;
#7068=ORIENTED_EDGE('',*,*,#4976,.F.) ;
#7069=ORIENTED_EDGE('',*,*,#5073,.T.) ;
#7070=ORIENTED_EDGE('',*,*,#5075,.T.) ;
#7071=ORIENTED_EDGE('',*,*,#5076,.F.) ;
#7072=ORIENTED_EDGE('',*,*,#4979,.F.) ;
#7073=ORIENTED_EDGE('',*,*,#5077,.F.) ;
#7074=ORIENTED_EDGE('',*,*,#5075,.F.) ;
#7075=ORIENTED_EDGE('',*,*,#5072,.T.) ;
#7076=ORIENTED_EDGE('',*,*,#5074,.T.) ;
#7077=ORIENTED_EDGE('',*,*,#4978,.F.) ;
#7078=ORIENTED_EDGE('',*,*,#5076,.T.) ;
#7079=ORIENTED_EDGE('',*,*,#5077,.T.) ;
#7080=ORIENTED_EDGE('',*,*,#4981,.F.) ;
#7081=ORIENTED_EDGE('',*,*,#5078,.T.) ;
#7082=ORIENTED_EDGE('',*,*,#4982,.F.) ;
#7083=ORIENTED_EDGE('',*,*,#5079,.F.) ;
#7084=ORIENTED_EDGE('',*,*,#4983,.F.) ;
#7085=ORIENTED_EDGE('',*,*,#5078,.F.) ;
#7086=ORIENTED_EDGE('',*,*,#4980,.F.) ;
#7087=ORIENTED_EDGE('',*,*,#5079,.T.) ;
#7088=ORIENTED_EDGE('',*,*,#4985,.F.) ;
#7089=ORIENTED_EDGE('',*,*,#5080,.T.) ;
#7090=ORIENTED_EDGE('',*,*,#4986,.F.) ;
#7091=ORIENTED_EDGE('',*,*,#5081,.F.) ;
#7092=ORIENTED_EDGE('',*,*,#4987,.F.) ;
#7093=ORIENTED_EDGE('',*,*,#5080,.F.) ;
#7094=ORIENTED_EDGE('',*,*,#4984,.F.) ;
#7095=ORIENTED_EDGE('',*,*,#5081,.T.) ;
#7096=ORIENTED_EDGE('',*,*,#4989,.F.) ;
#7097=ORIENTED_EDGE('',*,*,#5082,.T.) ;
#7098=ORIENTED_EDGE('',*,*,#4990,.F.) ;
#7099=ORIENTED_EDGE('',*,*,#5083,.F.) ;
#7100=ORIENTED_EDGE('',*,*,#4991,.F.) ;
#7101=ORIENTED_EDGE('',*,*,#5082,.F.) ;
#7102=ORIENTED_EDGE('',*,*,#4988,.F.) ;
#7103=ORIENTED_EDGE('',*,*,#5083,.T.) ;
#7104=ORIENTED_EDGE('',*,*,#4993,.F.) ;
#7105=ORIENTED_EDGE('',*,*,#5084,.T.) ;
#7106=ORIENTED_EDGE('',*,*,#4994,.F.) ;
#7107=ORIENTED_EDGE('',*,*,#5085,.F.) ;
#7108=ORIENTED_EDGE('',*,*,#5086,.F.) ;
#7109=ORIENTED_EDGE('',*,*,#4995,.F.) ;
#7110=ORIENTED_EDGE('',*,*,#5084,.F.) ;
#7111=ORIENTED_EDGE('',*,*,#4992,.F.) ;
#7112=ORIENTED_EDGE('',*,*,#5086,.T.) ;
#7113=ORIENTED_EDGE('',*,*,#5087,.T.) ;
#7114=ORIENTED_EDGE('',*,*,#5088,.F.) ;
#7115=ORIENTED_EDGE('',*,*,#5089,.F.) ;
#7116=ORIENTED_EDGE('',*,*,#4997,.F.) ;
#7117=ORIENTED_EDGE('',*,*,#5090,.F.) ;
#7118=ORIENTED_EDGE('',*,*,#5087,.F.) ;
#7119=ORIENTED_EDGE('',*,*,#5085,.T.) ;
#7120=ORIENTED_EDGE('',*,*,#4996,.F.) ;
#7121=ORIENTED_EDGE('',*,*,#5089,.T.) ;
#7122=ORIENTED_EDGE('',*,*,#5091,.T.) ;
#7123=ORIENTED_EDGE('',*,*,#5092,.F.) ;
#7124=ORIENTED_EDGE('',*,*,#4999,.F.) ;
#7125=ORIENTED_EDGE('',*,*,#5093,.F.) ;
#7126=ORIENTED_EDGE('',*,*,#5091,.F.) ;
#7127=ORIENTED_EDGE('',*,*,#5088,.T.) ;
#7128=ORIENTED_EDGE('',*,*,#5090,.T.) ;
#7129=ORIENTED_EDGE('',*,*,#4998,.F.) ;
#7130=ORIENTED_EDGE('',*,*,#5092,.T.) ;
#7131=ORIENTED_EDGE('',*,*,#5094,.T.) ;
#7132=ORIENTED_EDGE('',*,*,#5095,.F.) ;
#7133=ORIENTED_EDGE('',*,*,#5096,.F.) ;
#7134=ORIENTED_EDGE('',*,*,#5001,.F.) ;
#7135=ORIENTED_EDGE('',*,*,#5097,.F.) ;
#7136=ORIENTED_EDGE('',*,*,#5094,.F.) ;
#7137=ORIENTED_EDGE('',*,*,#5093,.T.) ;
#7138=ORIENTED_EDGE('',*,*,#5000,.F.) ;
#7139=ORIENTED_EDGE('',*,*,#5096,.T.) ;
#7140=ORIENTED_EDGE('',*,*,#5098,.T.) ;
#7141=ORIENTED_EDGE('',*,*,#5099,.F.) ;
#7142=ORIENTED_EDGE('',*,*,#5003,.F.) ;
#7143=ORIENTED_EDGE('',*,*,#5100,.F.) ;
#7144=ORIENTED_EDGE('',*,*,#5098,.F.) ;
#7145=ORIENTED_EDGE('',*,*,#5095,.T.) ;
#7146=ORIENTED_EDGE('',*,*,#5097,.T.) ;
#7147=ORIENTED_EDGE('',*,*,#5002,.F.) ;
#7148=ORIENTED_EDGE('',*,*,#5099,.T.) ;
#7149=ORIENTED_EDGE('',*,*,#5100,.T.) ;
#7150=ORIENTED_EDGE('',*,*,#5005,.F.) ;
#7151=ORIENTED_EDGE('',*,*,#5101,.T.) ;
#7152=ORIENTED_EDGE('',*,*,#5006,.F.) ;
#7153=ORIENTED_EDGE('',*,*,#5102,.F.) ;
#7154=ORIENTED_EDGE('',*,*,#5007,.F.) ;
#7155=ORIENTED_EDGE('',*,*,#5101,.F.) ;
#7156=ORIENTED_EDGE('',*,*,#5004,.F.) ;
#7157=ORIENTED_EDGE('',*,*,#5102,.T.) ;
#7158=ORIENTED_EDGE('',*,*,#5009,.F.) ;
#7159=ORIENTED_EDGE('',*,*,#5103,.T.) ;
#7160=ORIENTED_EDGE('',*,*,#5010,.F.) ;
#7161=ORIENTED_EDGE('',*,*,#5104,.F.) ;
#7162=ORIENTED_EDGE('',*,*,#5011,.F.) ;
#7163=ORIENTED_EDGE('',*,*,#5103,.F.) ;
#7164=ORIENTED_EDGE('',*,*,#5008,.F.) ;
#7165=ORIENTED_EDGE('',*,*,#5104,.T.) ;
#7166=ORIENTED_EDGE('',*,*,#5013,.F.) ;
#7167=ORIENTED_EDGE('',*,*,#5105,.T.) ;
#7168=ORIENTED_EDGE('',*,*,#5014,.F.) ;
#7169=ORIENTED_EDGE('',*,*,#5106,.F.) ;
#7170=ORIENTED_EDGE('',*,*,#5015,.F.) ;
#7171=ORIENTED_EDGE('',*,*,#5105,.F.) ;
#7172=ORIENTED_EDGE('',*,*,#5012,.F.) ;
#7173=ORIENTED_EDGE('',*,*,#5106,.T.) ;
#7174=ORIENTED_EDGE('',*,*,#5017,.F.) ;
#7175=ORIENTED_EDGE('',*,*,#5107,.T.) ;
#7176=ORIENTED_EDGE('',*,*,#5018,.F.) ;
#7177=ORIENTED_EDGE('',*,*,#5108,.F.) ;
#7178=ORIENTED_EDGE('',*,*,#5109,.F.) ;
#7179=ORIENTED_EDGE('',*,*,#5019,.F.) ;
#7180=ORIENTED_EDGE('',*,*,#5107,.F.) ;
#7181=ORIENTED_EDGE('',*,*,#5016,.F.) ;
#7182=ORIENTED_EDGE('',*,*,#5109,.T.) ;
#7183=ORIENTED_EDGE('',*,*,#5110,.T.) ;
#7184=ORIENTED_EDGE('',*,*,#5111,.F.) ;
#7185=ORIENTED_EDGE('',*,*,#5112,.F.) ;
#7186=ORIENTED_EDGE('',*,*,#5021,.F.) ;
#7187=ORIENTED_EDGE('',*,*,#5113,.F.) ;
#7188=ORIENTED_EDGE('',*,*,#5110,.F.) ;
#7189=ORIENTED_EDGE('',*,*,#5108,.T.) ;
#7190=ORIENTED_EDGE('',*,*,#5020,.F.) ;
#7191=ORIENTED_EDGE('',*,*,#5112,.T.) ;
#7192=ORIENTED_EDGE('',*,*,#5114,.T.) ;
#7193=ORIENTED_EDGE('',*,*,#5115,.F.) ;
#7194=ORIENTED_EDGE('',*,*,#5023,.F.) ;
#7195=ORIENTED_EDGE('',*,*,#5116,.F.) ;
#7196=ORIENTED_EDGE('',*,*,#5114,.F.) ;
#7197=ORIENTED_EDGE('',*,*,#5111,.T.) ;
#7198=ORIENTED_EDGE('',*,*,#5113,.T.) ;
#7199=ORIENTED_EDGE('',*,*,#5022,.F.) ;
#7200=ORIENTED_EDGE('',*,*,#5115,.T.) ;
#7201=ORIENTED_EDGE('',*,*,#5117,.T.) ;
#7202=ORIENTED_EDGE('',*,*,#5118,.F.) ;
#7203=ORIENTED_EDGE('',*,*,#5119,.F.) ;
#7204=ORIENTED_EDGE('',*,*,#5025,.F.) ;
#7205=ORIENTED_EDGE('',*,*,#5120,.F.) ;
#7206=ORIENTED_EDGE('',*,*,#5117,.F.) ;
#7207=ORIENTED_EDGE('',*,*,#5116,.T.) ;
#7208=ORIENTED_EDGE('',*,*,#5024,.F.) ;
#7209=ORIENTED_EDGE('',*,*,#5119,.T.) ;
#7210=ORIENTED_EDGE('',*,*,#5121,.T.) ;
#7211=ORIENTED_EDGE('',*,*,#5122,.F.) ;
#7212=ORIENTED_EDGE('',*,*,#5027,.F.) ;
#7213=ORIENTED_EDGE('',*,*,#5123,.F.) ;
#7214=ORIENTED_EDGE('',*,*,#5121,.F.) ;
#7215=ORIENTED_EDGE('',*,*,#5118,.T.) ;
#7216=ORIENTED_EDGE('',*,*,#5120,.T.) ;
#7217=ORIENTED_EDGE('',*,*,#5026,.F.) ;
#7218=ORIENTED_EDGE('',*,*,#5122,.T.) ;
#7219=ORIENTED_EDGE('',*,*,#5123,.T.) ;
#7220=ORIENTED_EDGE('',*,*,#5029,.F.) ;
#7221=ORIENTED_EDGE('',*,*,#5124,.T.) ;
#7222=ORIENTED_EDGE('',*,*,#5030,.F.) ;
#7223=ORIENTED_EDGE('',*,*,#5125,.F.) ;
#7224=ORIENTED_EDGE('',*,*,#5031,.F.) ;
#7225=ORIENTED_EDGE('',*,*,#5124,.F.) ;
#7226=ORIENTED_EDGE('',*,*,#5028,.F.) ;
#7227=ORIENTED_EDGE('',*,*,#5125,.T.) ;
#7228=ORIENTED_EDGE('',*,*,#5033,.F.) ;
#7229=ORIENTED_EDGE('',*,*,#5126,.T.) ;
#7230=ORIENTED_EDGE('',*,*,#5034,.F.) ;
#7231=ORIENTED_EDGE('',*,*,#5127,.F.) ;
#7232=ORIENTED_EDGE('',*,*,#5035,.F.) ;
#7233=ORIENTED_EDGE('',*,*,#5126,.F.) ;
#7234=ORIENTED_EDGE('',*,*,#5032,.F.) ;
#7235=ORIENTED_EDGE('',*,*,#5127,.T.) ;
#7236=ORIENTED_EDGE('',*,*,#5037,.F.) ;
#7237=ORIENTED_EDGE('',*,*,#5128,.T.) ;
#7238=ORIENTED_EDGE('',*,*,#5038,.F.) ;
#7239=ORIENTED_EDGE('',*,*,#5129,.F.) ;
#7240=ORIENTED_EDGE('',*,*,#5039,.F.) ;
#7241=ORIENTED_EDGE('',*,*,#5128,.F.) ;
#7242=ORIENTED_EDGE('',*,*,#5036,.F.) ;
#7243=ORIENTED_EDGE('',*,*,#5129,.T.) ;
#7244=ORIENTED_EDGE('',*,*,#5041,.F.) ;
#7245=ORIENTED_EDGE('',*,*,#5130,.T.) ;
#7246=ORIENTED_EDGE('',*,*,#5042,.F.) ;
#7247=ORIENTED_EDGE('',*,*,#5131,.F.) ;
#7248=ORIENTED_EDGE('',*,*,#5132,.F.) ;
#7249=ORIENTED_EDGE('',*,*,#5043,.F.) ;
#7250=ORIENTED_EDGE('',*,*,#5130,.F.) ;
#7251=ORIENTED_EDGE('',*,*,#5040,.F.) ;
#7252=ORIENTED_EDGE('',*,*,#5132,.T.) ;
#7253=ORIENTED_EDGE('',*,*,#5133,.T.) ;
#7254=ORIENTED_EDGE('',*,*,#5134,.F.) ;
#7255=ORIENTED_EDGE('',*,*,#5135,.F.) ;
#7256=ORIENTED_EDGE('',*,*,#5045,.F.) ;
#7257=ORIENTED_EDGE('',*,*,#5136,.F.) ;
#7258=ORIENTED_EDGE('',*,*,#5133,.F.) ;
#7259=ORIENTED_EDGE('',*,*,#5131,.T.) ;
#7260=ORIENTED_EDGE('',*,*,#5044,.F.) ;
#7261=ORIENTED_EDGE('',*,*,#5135,.T.) ;
#7262=ORIENTED_EDGE('',*,*,#5137,.T.) ;
#7263=ORIENTED_EDGE('',*,*,#5138,.F.) ;
#7264=ORIENTED_EDGE('',*,*,#5137,.F.) ;
#7265=ORIENTED_EDGE('',*,*,#5134,.T.) ;
#7266=ORIENTED_EDGE('',*,*,#5136,.T.) ;
#7267=ORIENTED_EDGE('',*,*,#5046,.F.) ;
#7268=ORIENTED_EDGE('',*,*,#5138,.T.) ;
#7693=PLANE('',#9679) ;
#7694=PLANE('',#9767) ;
#8111=ADVANCED_FACE('',(#1724),#260,.T.) ;
#8112=ADVANCED_FACE('',(#1725),#261,.T.) ;
#8113=ADVANCED_FACE('',(#1726),#262,.T.) ;
#8114=ADVANCED_FACE('',(#1727),#263,.T.) ;
#8115=ADVANCED_FACE('',(#1728),#264,.T.) ;
#8116=ADVANCED_FACE('',(#1729),#265,.T.) ;
#8117=ADVANCED_FACE('',(#1730),#266,.T.) ;
#8118=ADVANCED_FACE('',(#1731),#267,.T.) ;
#8119=ADVANCED_FACE('',(#1732),#268,.T.) ;
#8120=ADVANCED_FACE('',(#1733),#269,.T.) ;
#8121=ADVANCED_FACE('',(#1734),#270,.T.) ;
#8122=ADVANCED_FACE('',(#1735),#271,.T.) ;
#8123=ADVANCED_FACE('',(#1736),#272,.T.) ;
#8124=ADVANCED_FACE('',(#1737),#273,.T.) ;
#8125=ADVANCED_FACE('',(#1738),#274,.T.) ;
#8126=ADVANCED_FACE('',(#1739),#275,.T.) ;
#8127=ADVANCED_FACE('',(#1740),#276,.T.) ;
#8128=ADVANCED_FACE('',(#1741),#277,.T.) ;
#8129=ADVANCED_FACE('',(#1742),#278,.T.) ;
#8130=ADVANCED_FACE('',(#1743),#279,.T.) ;
#8131=ADVANCED_FACE('',(#1744),#280,.T.) ;
#8132=ADVANCED_FACE('',(#1745),#281,.T.) ;
#8133=ADVANCED_FACE('',(#1746),#282,.T.) ;
#8134=ADVANCED_FACE('',(#1747),#283,.T.) ;
#8135=ADVANCED_FACE('',(#1748),#284,.T.) ;
#8136=ADVANCED_FACE('',(#1749),#285,.T.) ;
#8137=ADVANCED_FACE('',(#1750),#286,.T.) ;
#8138=ADVANCED_FACE('',(#1751),#287,.T.) ;
#8139=ADVANCED_FACE('',(#1752),#288,.T.) ;
#8140=ADVANCED_FACE('',(#1753),#289,.T.) ;
#8141=ADVANCED_FACE('',(#1754),#290,.T.) ;
#8142=ADVANCED_FACE('',(#1755),#761,.T.) ;
#8143=ADVANCED_FACE('',(#1756),#7693,.T.) ;
#8144=ADVANCED_FACE('',(#1757),#762,.T.) ;
#8145=ADVANCED_FACE('',(#1758),#763,.T.) ;
#8146=ADVANCED_FACE('',(#1759),#764,.T.) ;
#8147=ADVANCED_FACE('',(#1760),#765,.T.) ;
#8148=ADVANCED_FACE('',(#1761),#766,.T.) ;
#8149=ADVANCED_FACE('',(#1762),#767,.T.) ;
#8150=ADVANCED_FACE('',(#1763),#768,.T.) ;
#8151=ADVANCED_FACE('',(#1764),#769,.T.) ;
#8152=ADVANCED_FACE('',(#1765),#770,.T.) ;
#8153=ADVANCED_FACE('',(#1766),#771,.T.) ;
#8154=ADVANCED_FACE('',(#1767),#772,.T.) ;
#8155=ADVANCED_FACE('',(#1768),#773,.T.) ;
#8156=ADVANCED_FACE('',(#1769),#774,.T.) ;
#8157=ADVANCED_FACE('',(#1770),#775,.T.) ;
#8158=ADVANCED_FACE('',(#1771),#776,.T.) ;
#8159=ADVANCED_FACE('',(#1772),#777,.T.) ;
#8160=ADVANCED_FACE('',(#1773),#778,.T.) ;
#8161=ADVANCED_FACE('',(#1774),#779,.T.) ;
#8162=ADVANCED_FACE('',(#1775),#780,.T.) ;
#8163=ADVANCED_FACE('',(#1776),#781,.T.) ;
#8164=ADVANCED_FACE('',(#1777),#782,.T.) ;
#8165=ADVANCED_FACE('',(#1778),#783,.T.) ;
#8166=ADVANCED_FACE('',(#1779),#784,.T.) ;
#8167=ADVANCED_FACE('',(#1780),#785,.T.) ;
#8168=ADVANCED_FACE('',(#1781),#786,.T.) ;
#8169=ADVANCED_FACE('',(#1782),#787,.T.) ;
#8170=ADVANCED_FACE('',(#1783),#788,.T.) ;
#8171=ADVANCED_FACE('',(#1784),#789,.T.) ;
#8172=ADVANCED_FACE('',(#1785),#790,.T.) ;
#8173=ADVANCED_FACE('',(#1786),#791,.T.) ;
#8174=ADVANCED_FACE('',(#1787),#792,.T.) ;
#8175=ADVANCED_FACE('',(#1788),#7694,.T.) ;
#8280=CLOSED_SHELL('',(#8111,#8112,#8113,#8114,#8115,#8116,#8117,#8118,
#8119,#8120,#8121,#8122,#8123,#8124,#8125,#8126,#8127,#8128,#8129,#8130,
#8131,#8132,#8133,#8134,#8135,#8136,#8137,#8138,#8139,#8140,#8141,#8142,
#8143,#8144,#8145,#8146,#8147,#8148,#8149,#8150,#8151,#8152,#8153,#8154,
#8155,#8156,#8157,#8158,#8159,#8160,#8161,#8162,#8163,#8164,#8165,#8166,
#8167,#8168,#8169,#8170,#8171,#8172,#8173,#8174,#8175)) ;
#9548=AXIS2_PLACEMENT_3D('',#14684,#12005,#12006) ;
#9549=AXIS2_PLACEMENT_3D('',#14685,#12007,#12008) ;
#9550=AXIS2_PLACEMENT_3D('',#14688,#12009,#12010) ;
#9551=AXIS2_PLACEMENT_3D('',#14689,#12011,#12012) ;
#9552=AXIS2_PLACEMENT_3D('',#14690,#12013,#12014) ;
#9553=AXIS2_PLACEMENT_3D('',#14693,#12015,#12016) ;
#9554=AXIS2_PLACEMENT_3D('',#14695,#12017,#12018) ;
#9555=AXIS2_PLACEMENT_3D('',#14696,#12019,#12020) ;
#9556=AXIS2_PLACEMENT_3D('',#14697,#12021,#12022) ;
#9557=AXIS2_PLACEMENT_3D('',#14700,#12023,#12024) ;
#9558=AXIS2_PLACEMENT_3D('',#14702,#12025,#12026) ;
#9559=AXIS2_PLACEMENT_3D('',#14704,#12027,#12028) ;
#9560=AXIS2_PLACEMENT_3D('',#14705,#12029,#12030) ;
#9561=AXIS2_PLACEMENT_3D('',#14706,#12031,#12032) ;
#9562=AXIS2_PLACEMENT_3D('',#14709,#12033,#12034) ;
#9563=AXIS2_PLACEMENT_3D('',#14711,#12035,#12036) ;
#9564=AXIS2_PLACEMENT_3D('',#14713,#12037,#12038) ;
#9565=AXIS2_PLACEMENT_3D('',#14714,#12039,#12040) ;
#9566=AXIS2_PLACEMENT_3D('',#14715,#12041,#12042) ;
#9567=AXIS2_PLACEMENT_3D('',#14718,#12043,#12044) ;
#9568=AXIS2_PLACEMENT_3D('',#14720,#12045,#12046) ;
#9569=AXIS2_PLACEMENT_3D('',#14722,#12047,#12048) ;
#9570=AXIS2_PLACEMENT_3D('',#14723,#12049,#12050) ;
#9571=AXIS2_PLACEMENT_3D('',#14724,#12051,#12052) ;
#9572=AXIS2_PLACEMENT_3D('',#14727,#12053,#12054) ;
#9573=AXIS2_PLACEMENT_3D('',#14729,#12055,#12056) ;
#9574=AXIS2_PLACEMENT_3D('',#14730,#12057,#12058) ;
#9575=AXIS2_PLACEMENT_3D('',#14731,#12059,#12060) ;
#9576=AXIS2_PLACEMENT_3D('',#14734,#12061,#12062) ;
#9577=AXIS2_PLACEMENT_3D('',#14735,#12063,#12064) ;
#9578=AXIS2_PLACEMENT_3D('',#14736,#12065,#12066) ;
#9579=AXIS2_PLACEMENT_3D('',#14739,#12067,#12068) ;
#9580=AXIS2_PLACEMENT_3D('',#14740,#12069,#12070) ;
#9581=AXIS2_PLACEMENT_3D('',#14741,#12071,#12072) ;
#9582=AXIS2_PLACEMENT_3D('',#14744,#12073,#12074) ;
#9583=AXIS2_PLACEMENT_3D('',#14745,#12075,#12076) ;
#9584=AXIS2_PLACEMENT_3D('',#14746,#12077,#12078) ;
#9585=AXIS2_PLACEMENT_3D('',#14749,#12079,#12080) ;
#9586=AXIS2_PLACEMENT_3D('',#14751,#12081,#12082) ;
#9587=AXIS2_PLACEMENT_3D('',#14752,#12083,#12084) ;
#9588=AXIS2_PLACEMENT_3D('',#14753,#12085,#12086) ;
#9589=AXIS2_PLACEMENT_3D('',#14756,#12087,#12088) ;
#9590=AXIS2_PLACEMENT_3D('',#14758,#12089,#12090) ;
#9591=AXIS2_PLACEMENT_3D('',#14760,#12091,#12092) ;
#9592=AXIS2_PLACEMENT_3D('',#14761,#12093,#12094) ;
#9593=AXIS2_PLACEMENT_3D('',#14762,#12095,#12096) ;
#9594=AXIS2_PLACEMENT_3D('',#14765,#12097,#12098) ;
#9595=AXIS2_PLACEMENT_3D('',#14767,#12099,#12100) ;
#9596=AXIS2_PLACEMENT_3D('',#14769,#12101,#12102) ;
#9597=AXIS2_PLACEMENT_3D('',#14770,#12103,#12104) ;
#9598=AXIS2_PLACEMENT_3D('',#14771,#12105,#12106) ;
#9599=AXIS2_PLACEMENT_3D('',#14774,#12107,#12108) ;
#9600=AXIS2_PLACEMENT_3D('',#14776,#12109,#12110) ;
#9601=AXIS2_PLACEMENT_3D('',#14778,#12111,#12112) ;
#9602=AXIS2_PLACEMENT_3D('',#14779,#12113,#12114) ;
#9603=AXIS2_PLACEMENT_3D('',#14780,#12115,#12116) ;
#9604=AXIS2_PLACEMENT_3D('',#14783,#12117,#12118) ;
#9605=AXIS2_PLACEMENT_3D('',#14785,#12119,#12120) ;
#9606=AXIS2_PLACEMENT_3D('',#14786,#12121,#12122) ;
#9607=AXIS2_PLACEMENT_3D('',#14787,#12123,#12124) ;
#9608=AXIS2_PLACEMENT_3D('',#14790,#12125,#12126) ;
#9609=AXIS2_PLACEMENT_3D('',#14791,#12127,#12128) ;
#9610=AXIS2_PLACEMENT_3D('',#14792,#12129,#12130) ;
#9611=AXIS2_PLACEMENT_3D('',#14795,#12131,#12132) ;
#9612=AXIS2_PLACEMENT_3D('',#14796,#12133,#12134) ;
#9613=AXIS2_PLACEMENT_3D('',#14797,#12135,#12136) ;
#9614=AXIS2_PLACEMENT_3D('',#14800,#12137,#12138) ;
#9615=AXIS2_PLACEMENT_3D('',#14801,#12139,#12140) ;
#9616=AXIS2_PLACEMENT_3D('',#14802,#12141,#12142) ;
#9617=AXIS2_PLACEMENT_3D('',#14805,#12143,#12144) ;
#9618=AXIS2_PLACEMENT_3D('',#14807,#12145,#12146) ;
#9619=AXIS2_PLACEMENT_3D('',#14808,#12147,#12148) ;
#9620=AXIS2_PLACEMENT_3D('',#14809,#12149,#12150) ;
#9621=AXIS2_PLACEMENT_3D('',#14812,#12151,#12152) ;
#9622=AXIS2_PLACEMENT_3D('',#14814,#12153,#12154) ;
#9623=AXIS2_PLACEMENT_3D('',#14816,#12155,#12156) ;
#9624=AXIS2_PLACEMENT_3D('',#14817,#12157,#12158) ;
#9625=AXIS2_PLACEMENT_3D('',#14818,#12159,#12160) ;
#9626=AXIS2_PLACEMENT_3D('',#14821,#12161,#12162) ;
#9627=AXIS2_PLACEMENT_3D('',#14823,#12163,#12164) ;
#9628=AXIS2_PLACEMENT_3D('',#14825,#12165,#12166) ;
#9629=AXIS2_PLACEMENT_3D('',#14826,#12167,#12168) ;
#9630=AXIS2_PLACEMENT_3D('',#14827,#12169,#12170) ;
#9631=AXIS2_PLACEMENT_3D('',#14830,#12171,#12172) ;
#9632=AXIS2_PLACEMENT_3D('',#14832,#12173,#12174) ;
#9633=AXIS2_PLACEMENT_3D('',#14834,#12175,#12176) ;
#9634=AXIS2_PLACEMENT_3D('',#14835,#12177,#12178) ;
#9635=AXIS2_PLACEMENT_3D('',#14836,#12179,#12180) ;
#9636=AXIS2_PLACEMENT_3D('',#14839,#12181,#12182) ;
#9637=AXIS2_PLACEMENT_3D('',#14841,#12183,#12184) ;
#9638=AXIS2_PLACEMENT_3D('',#14842,#12185,#12186) ;
#9639=AXIS2_PLACEMENT_3D('',#14843,#12187,#12188) ;
#9640=AXIS2_PLACEMENT_3D('',#14846,#12189,#12190) ;
#9641=AXIS2_PLACEMENT_3D('',#14847,#12191,#12192) ;
#9642=AXIS2_PLACEMENT_3D('',#14848,#12193,#12194) ;
#9643=AXIS2_PLACEMENT_3D('',#14851,#12195,#12196) ;
#9644=AXIS2_PLACEMENT_3D('',#14852,#12197,#12198) ;
#9645=AXIS2_PLACEMENT_3D('',#14853,#12199,#12200) ;
#9646=AXIS2_PLACEMENT_3D('',#14856,#12201,#12202) ;
#9647=AXIS2_PLACEMENT_3D('',#14857,#12203,#12204) ;
#9648=AXIS2_PLACEMENT_3D('',#14858,#12205,#12206) ;
#9649=AXIS2_PLACEMENT_3D('',#14861,#12207,#12208) ;
#9650=AXIS2_PLACEMENT_3D('',#14863,#12209,#12210) ;
#9651=AXIS2_PLACEMENT_3D('',#14864,#12211,#12212) ;
#9652=AXIS2_PLACEMENT_3D('',#14865,#12213,#12214) ;
#9653=AXIS2_PLACEMENT_3D('',#14868,#12215,#12216) ;
#9654=AXIS2_PLACEMENT_3D('',#14870,#12217,#12218) ;
#9655=AXIS2_PLACEMENT_3D('',#14872,#12219,#12220) ;
#9656=AXIS2_PLACEMENT_3D('',#14873,#12221,#12222) ;
#9657=AXIS2_PLACEMENT_3D('',#14874,#12223,#12224) ;
#9658=AXIS2_PLACEMENT_3D('',#14877,#12225,#12226) ;
#9659=AXIS2_PLACEMENT_3D('',#14879,#12227,#12228) ;
#9660=AXIS2_PLACEMENT_3D('',#14881,#12229,#12230) ;
#9661=AXIS2_PLACEMENT_3D('',#14882,#12231,#12232) ;
#9662=AXIS2_PLACEMENT_3D('',#14883,#12233,#12234) ;
#9663=AXIS2_PLACEMENT_3D('',#14886,#12235,#12236) ;
#9664=AXIS2_PLACEMENT_3D('',#14888,#12237,#12238) ;
#9665=AXIS2_PLACEMENT_3D('',#14890,#12239,#12240) ;
#9666=AXIS2_PLACEMENT_3D('',#14891,#12241,#12242) ;
#9667=AXIS2_PLACEMENT_3D('',#14892,#12243,#12244) ;
#9668=AXIS2_PLACEMENT_3D('',#14895,#12245,#12246) ;
#9669=AXIS2_PLACEMENT_3D('',#14897,#12247,#12248) ;
#9670=AXIS2_PLACEMENT_3D('',#14898,#12249,#12250) ;
#9671=AXIS2_PLACEMENT_3D('',#14899,#12251,#12252) ;
#9672=AXIS2_PLACEMENT_3D('',#14902,#12253,#12254) ;
#9673=AXIS2_PLACEMENT_3D('',#14903,#12255,#12256) ;
#9674=AXIS2_PLACEMENT_3D('',#14904,#12257,#12258) ;
#9675=AXIS2_PLACEMENT_3D('',#14906,#12259,#12260) ;
#9676=AXIS2_PLACEMENT_3D('',#14910,#12262,#12263) ;
#9677=AXIS2_PLACEMENT_3D('',#14911,#12264,#12265) ;
#9678=AXIS2_PLACEMENT_3D('',#14912,#12266,#12267) ;
#9679=AXIS2_PLACEMENT_3D('',#14913,#12268,#12269) ;
#9680=AXIS2_PLACEMENT_3D('',#14914,#12270,#12271) ;
#9681=AXIS2_PLACEMENT_3D('',#14917,#12273,#12274) ;
#9682=AXIS2_PLACEMENT_3D('',#14918,#12275,#12276) ;
#9683=AXIS2_PLACEMENT_3D('',#14919,#12277,#12278) ;
#9684=AXIS2_PLACEMENT_3D('',#14921,#12280,#12281) ;
#9685=AXIS2_PLACEMENT_3D('',#14922,#12282,#12283) ;
#9686=AXIS2_PLACEMENT_3D('',#14924,#12285,#12286) ;
#9687=AXIS2_PLACEMENT_3D('',#14925,#12287,#12288) ;
#9688=AXIS2_PLACEMENT_3D('',#14927,#12290,#12291) ;
#9689=AXIS2_PLACEMENT_3D('',#14928,#12292,#12293) ;
#9690=AXIS2_PLACEMENT_3D('',#14931,#12295,#12296) ;
#9691=AXIS2_PLACEMENT_3D('',#14932,#12297,#12298) ;
#9692=AXIS2_PLACEMENT_3D('',#14933,#12299,#12300) ;
#9693=AXIS2_PLACEMENT_3D('',#14937,#12302,#12303) ;
#9694=AXIS2_PLACEMENT_3D('',#14938,#12304,#12305) ;
#9695=AXIS2_PLACEMENT_3D('',#14939,#12306,#12307) ;
#9696=AXIS2_PLACEMENT_3D('',#14940,#12308,#12309) ;
#9697=AXIS2_PLACEMENT_3D('',#14943,#12311,#12312) ;
#9698=AXIS2_PLACEMENT_3D('',#14944,#12313,#12314) ;
#9699=AXIS2_PLACEMENT_3D('',#14945,#12315,#12316) ;
#9700=AXIS2_PLACEMENT_3D('',#14949,#12318,#12319) ;
#9701=AXIS2_PLACEMENT_3D('',#14950,#12320,#12321) ;
#9702=AXIS2_PLACEMENT_3D('',#14951,#12322,#12323) ;
#9703=AXIS2_PLACEMENT_3D('',#14952,#12324,#12325) ;
#9704=AXIS2_PLACEMENT_3D('',#14955,#12327,#12328) ;
#9705=AXIS2_PLACEMENT_3D('',#14956,#12329,#12330) ;
#9706=AXIS2_PLACEMENT_3D('',#14957,#12331,#12332) ;
#9707=AXIS2_PLACEMENT_3D('',#14959,#12334,#12335) ;
#9708=AXIS2_PLACEMENT_3D('',#14960,#12336,#12337) ;
#9709=AXIS2_PLACEMENT_3D('',#14962,#12339,#12340) ;
#9710=AXIS2_PLACEMENT_3D('',#14963,#12341,#12342) ;
#9711=AXIS2_PLACEMENT_3D('',#14965,#12344,#12345) ;
#9712=AXIS2_PLACEMENT_3D('',#14966,#12346,#12347) ;
#9713=AXIS2_PLACEMENT_3D('',#14969,#12349,#12350) ;
#9714=AXIS2_PLACEMENT_3D('',#14970,#12351,#12352) ;
#9715=AXIS2_PLACEMENT_3D('',#14971,#12353,#12354) ;
#9716=AXIS2_PLACEMENT_3D('',#14975,#12356,#12357) ;
#9717=AXIS2_PLACEMENT_3D('',#14976,#12358,#12359) ;
#9718=AXIS2_PLACEMENT_3D('',#14977,#12360,#12361) ;
#9719=AXIS2_PLACEMENT_3D('',#14978,#12362,#12363) ;
#9720=AXIS2_PLACEMENT_3D('',#14981,#12365,#12366) ;
#9721=AXIS2_PLACEMENT_3D('',#14982,#12367,#12368) ;
#9722=AXIS2_PLACEMENT_3D('',#14983,#12369,#12370) ;
#9723=AXIS2_PLACEMENT_3D('',#14987,#12372,#12373) ;
#9724=AXIS2_PLACEMENT_3D('',#14988,#12374,#12375) ;
#9725=AXIS2_PLACEMENT_3D('',#14989,#12376,#12377) ;
#9726=AXIS2_PLACEMENT_3D('',#14990,#12378,#12379) ;
#9727=AXIS2_PLACEMENT_3D('',#14993,#12381,#12382) ;
#9728=AXIS2_PLACEMENT_3D('',#14994,#12383,#12384) ;
#9729=AXIS2_PLACEMENT_3D('',#14995,#12385,#12386) ;
#9730=AXIS2_PLACEMENT_3D('',#14997,#12388,#12389) ;
#9731=AXIS2_PLACEMENT_3D('',#14998,#12390,#12391) ;
#9732=AXIS2_PLACEMENT_3D('',#15000,#12393,#12394) ;
#9733=AXIS2_PLACEMENT_3D('',#15001,#12395,#12396) ;
#9734=AXIS2_PLACEMENT_3D('',#15003,#12398,#12399) ;
#9735=AXIS2_PLACEMENT_3D('',#15004,#12400,#12401) ;
#9736=AXIS2_PLACEMENT_3D('',#15007,#12403,#12404) ;
#9737=AXIS2_PLACEMENT_3D('',#15008,#12405,#12406) ;
#9738=AXIS2_PLACEMENT_3D('',#15009,#12407,#12408) ;
#9739=AXIS2_PLACEMENT_3D('',#15013,#12410,#12411) ;
#9740=AXIS2_PLACEMENT_3D('',#15014,#12412,#12413) ;
#9741=AXIS2_PLACEMENT_3D('',#15015,#12414,#12415) ;
#9742=AXIS2_PLACEMENT_3D('',#15016,#12416,#12417) ;
#9743=AXIS2_PLACEMENT_3D('',#15019,#12419,#12420) ;
#9744=AXIS2_PLACEMENT_3D('',#15020,#12421,#12422) ;
#9745=AXIS2_PLACEMENT_3D('',#15021,#12423,#12424) ;
#9746=AXIS2_PLACEMENT_3D('',#15025,#12426,#12427) ;
#9747=AXIS2_PLACEMENT_3D('',#15026,#12428,#12429) ;
#9748=AXIS2_PLACEMENT_3D('',#15027,#12430,#12431) ;
#9749=AXIS2_PLACEMENT_3D('',#15028,#12432,#12433) ;
#9750=AXIS2_PLACEMENT_3D('',#15031,#12435,#12436) ;
#9751=AXIS2_PLACEMENT_3D('',#15032,#12437,#12438) ;
#9752=AXIS2_PLACEMENT_3D('',#15033,#12439,#12440) ;
#9753=AXIS2_PLACEMENT_3D('',#15035,#12442,#12443) ;
#9754=AXIS2_PLACEMENT_3D('',#15036,#12444,#12445) ;
#9755=AXIS2_PLACEMENT_3D('',#15038,#12447,#12448) ;
#9756=AXIS2_PLACEMENT_3D('',#15039,#12449,#12450) ;
#9757=AXIS2_PLACEMENT_3D('',#15041,#12452,#12453) ;
#9758=AXIS2_PLACEMENT_3D('',#15042,#12454,#12455) ;
#9759=AXIS2_PLACEMENT_3D('',#15045,#12457,#12458) ;
#9760=AXIS2_PLACEMENT_3D('',#15046,#12459,#12460) ;
#9761=AXIS2_PLACEMENT_3D('',#15047,#12461,#12462) ;
#9762=AXIS2_PLACEMENT_3D('',#15051,#12464,#12465) ;
#9763=AXIS2_PLACEMENT_3D('',#15052,#12466,#12467) ;
#9764=AXIS2_PLACEMENT_3D('',#15053,#12468,#12469) ;
#9765=AXIS2_PLACEMENT_3D('',#15054,#12470,#12471) ;
#9766=AXIS2_PLACEMENT_3D('',#15057,#12473,#12474) ;
#9767=AXIS2_PLACEMENT_3D('',#15058,#12475,#12476) ;
#12005=DIRECTION('axis',(0.,0.,1.)) ;
#12006=DIRECTION('refdir',(1.,0.,0.)) ;
#12007=DIRECTION('center_axis',(0.,0.,1.)) ;
#12008=DIRECTION('ref_axis',(1.,0.,0.)) ;
#12009=DIRECTION('center_axis',(-0.381869435050518,-0.921914369154711,-0.0651891902102614)) ;
#12010=DIRECTION('ref_axis',(0.924216281275221,-0.38091832663704,-0.0269349931843283)) ;
#12011=DIRECTION('center_axis',(0.921914369154713,0.381869435050514,0.0651891902102614)) ;
#12012=DIRECTION('ref_axis',(0.38739372213043,-0.908767745068236,-0.155136358012961)) ;
#12013=DIRECTION('center_axis',(0.,0.,1.)) ;
#12014=DIRECTION('ref_axis',(1.,0.,0.)) ;
#12015=DIRECTION('center_axis',(-0.921914369154713,-0.381869435050514,-0.0651891902102614)) ;
#12016=DIRECTION('ref_axis',(0.38739372213043,-0.908767745068236,-0.155136358012961)) ;
#12017=DIRECTION('center_axis',(0.921914369154711,-0.381869435050519,0.0651891902102617)) ;
#12018=DIRECTION('ref_axis',(0.387393722130434,0.908767745068234,-0.155136358012959)) ;
#12019=DIRECTION('center_axis',(0.921914369154711,-0.381869435050519,0.0651891902102617)) ;
#12020=DIRECTION('ref_axis',(0.387393722130434,0.908767745068234,-0.155136358012959)) ;
#12021=DIRECTION('center_axis',(0.,0.,1.)) ;
#12022=DIRECTION('ref_axis',(-0.707106781186548,-0.707106781186548,0.)) ;
#12023=DIRECTION('center_axis',(-0.921914369154711,0.381869435050519,-0.0651891902102617)) ;
#12024=DIRECTION('ref_axis',(0.387393722130434,0.908767745068234,-0.155136358012959)) ;
#12025=DIRECTION('center_axis',(-0.921914369154711,0.381869435050519,-0.0651891902102617)) ;
#12026=DIRECTION('ref_axis',(0.387393722130434,0.908767745068234,-0.155136358012959)) ;
#12027=DIRECTION('center_axis',(0.381869435050516,-0.921914369154712,0.0651891902102615)) ;
#12028=DIRECTION('ref_axis',(0.924216281275222,0.380918326637037,-0.0269349931843281)) ;
#12029=DIRECTION('center_axis',(0.381869435050516,-0.921914369154712,0.0651891902102615)) ;
#12030=DIRECTION('ref_axis',(0.924216281275222,0.380918326637037,-0.0269349931843281)) ;
#12031=DIRECTION('center_axis',(0.,0.,1.)) ;
#12032=DIRECTION('ref_axis',(-1.,0.,0.)) ;
#12033=DIRECTION('center_axis',(-0.381869435050516,0.921914369154712,-0.0651891902102615)) ;
#12034=DIRECTION('ref_axis',(0.924216281275222,0.380918326637037,-0.0269349931843281)) ;
#12035=DIRECTION('center_axis',(-0.381869435050516,0.921914369154712,-0.0651891902102615)) ;
#12036=DIRECTION('ref_axis',(0.924216281275222,0.380918326637037,-0.0269349931843281)) ;
#12037=DIRECTION('center_axis',(-0.381869435050518,-0.921914369154711,0.0651891902102613)) ;
#12038=DIRECTION('ref_axis',(0.924216281275221,-0.380918326637039,0.0269349931843282)) ;
#12039=DIRECTION('center_axis',(-0.381869435050518,-0.921914369154711,0.0651891902102613)) ;
#12040=DIRECTION('ref_axis',(0.924216281275221,-0.380918326637039,0.0269349931843282)) ;
#12041=DIRECTION('center_axis',(0.,0.,1.)) ;
#12042=DIRECTION('ref_axis',(-0.707106781186509,0.707106781186586,0.)) ;
#12043=DIRECTION('center_axis',(0.381869435050518,0.921914369154711,-0.0651891902102613)) ;
#12044=DIRECTION('ref_axis',(0.924216281275221,-0.380918326637039,0.0269349931843282)) ;
#12045=DIRECTION('center_axis',(0.381869435050518,0.921914369154711,-0.0651891902102613)) ;
#12046=DIRECTION('ref_axis',(0.924216281275221,-0.380918326637039,0.0269349931843282)) ;
#12047=DIRECTION('center_axis',(-0.921914369154711,-0.381869435050517,0.0651891902102618)) ;
#12048=DIRECTION('ref_axis',(0.387393722130432,-0.908767745068235,0.15513635801296)) ;
#12049=DIRECTION('center_axis',(-0.921914369154711,-0.381869435050517,0.0651891902102618)) ;
#12050=DIRECTION('ref_axis',(0.387393722130432,-0.908767745068235,0.15513635801296)) ;
#12051=DIRECTION('center_axis',(0.,0.,1.)) ;
#12052=DIRECTION('ref_axis',(1.,0.,0.)) ;
#12053=DIRECTION('center_axis',(0.921914369154711,0.381869435050517,-0.0651891902102618)) ;
#12054=DIRECTION('ref_axis',(0.387393722130432,-0.908767745068235,0.15513635801296)) ;
#12055=DIRECTION('center_axis',(0.921914369154711,0.381869435050517,-0.0651891902102618)) ;
#12056=DIRECTION('ref_axis',(0.387393722130432,-0.908767745068235,0.15513635801296)) ;
#12057=DIRECTION('center_axis',(-0.921914369154711,0.381869435050517,0.0651891902102614)) ;
#12058=DIRECTION('ref_axis',(0.387393722130432,0.908767745068235,0.155136358012959)) ;
#12059=DIRECTION('center_axis',(0.,0.,1.)) ;
#12060=DIRECTION('ref_axis',(1.,0.,0.)) ;
#12061=DIRECTION('center_axis',(0.921914369154711,-0.381869435050517,-0.0651891902102614)) ;
#12062=DIRECTION('ref_axis',(0.387393722130432,0.908767745068235,0.155136358012959)) ;
#12063=DIRECTION('center_axis',(-0.381869435050518,0.921914369154711,0.0651891902102615)) ;
#12064=DIRECTION('ref_axis',(0.924216281275221,0.380918326637039,0.0269349931843283)) ;
#12065=DIRECTION('center_axis',(0.,0.,1.)) ;
#12066=DIRECTION('ref_axis',(1.,0.,0.)) ;
#12067=DIRECTION('center_axis',(0.381869435050518,-0.921914369154711,-0.0651891902102615)) ;
#12068=DIRECTION('ref_axis',(0.924216281275221,0.380918326637039,0.0269349931843283)) ;
#12069=DIRECTION('center_axis',(0.381869435050518,0.921914369154711,0.0651891902102614)) ;
#12070=DIRECTION('ref_axis',(0.924216281275221,-0.38091832663704,-0.0269349931843283)) ;
#12071=DIRECTION('center_axis',(0.,0.,1.)) ;
#12072=DIRECTION('ref_axis',(1.,0.,0.)) ;
#12073=DIRECTION('center_axis',(-0.381869435050518,-0.921914369154711,-0.0651891902102614)) ;
#12074=DIRECTION('ref_axis',(0.924216281275221,-0.38091832663704,-0.0269349931843283)) ;
#12075=DIRECTION('center_axis',(0.921914369154711,0.381869435050517,0.0651891902102614)) ;
#12076=DIRECTION('ref_axis',(0.387393722130433,-0.908767745068235,-0.155136358012959)) ;
#12077=DIRECTION('center_axis',(0.,0.,1.)) ;
#12078=DIRECTION('ref_axis',(1.,0.,0.)) ;
#12079=DIRECTION('center_axis',(-0.921914369154711,-0.381869435050517,-0.0651891902102614)) ;
#12080=DIRECTION('ref_axis',(0.387393722130433,-0.908767745068235,-0.155136358012959)) ;
#12081=DIRECTION('center_axis',(0.921914369154711,-0.381869435050518,0.0651891902102616)) ;
#12082=DIRECTION('ref_axis',(0.387393722130434,0.908767745068234,-0.155136358012959)) ;
#12083=DIRECTION('center_axis',(0.921914369154711,-0.381869435050518,0.0651891902102616)) ;
#12084=DIRECTION('ref_axis',(0.387393722130434,0.908767745068234,-0.155136358012959)) ;
#12085=DIRECTION('center_axis',(0.,0.,1.)) ;
#12086=DIRECTION('ref_axis',(-0.707106781186703,-0.707106781186392,0.)) ;
#12087=DIRECTION('center_axis',(-0.921914369154711,0.381869435050518,-0.0651891902102616)) ;
#12088=DIRECTION('ref_axis',(0.387393722130434,0.908767745068234,-0.155136358012959)) ;
#12089=DIRECTION('center_axis',(-0.921914369154711,0.381869435050518,-0.0651891902102616)) ;
#12090=DIRECTION('ref_axis',(0.387393722130434,0.908767745068234,-0.155136358012959)) ;
#12091=DIRECTION('center_axis',(0.381869435050516,-0.921914369154712,0.0651891902102615)) ;
#12092=DIRECTION('ref_axis',(0.924216281275222,0.380918326637037,-0.0269349931843281)) ;
#12093=DIRECTION('center_axis',(0.381869435050516,-0.921914369154712,0.0651891902102615)) ;
#12094=DIRECTION('ref_axis',(0.924216281275222,0.380918326637037,-0.0269349931843281)) ;
#12095=DIRECTION('center_axis',(0.,0.,1.)) ;
#12096=DIRECTION('ref_axis',(-1.,1.55431223447522E-13,0.)) ;
#12097=DIRECTION('center_axis',(-0.381869435050516,0.921914369154712,-0.0651891902102615)) ;
#12098=DIRECTION('ref_axis',(0.924216281275222,0.380918326637037,-0.0269349931843281)) ;
#12099=DIRECTION('center_axis',(-0.381869435050516,0.921914369154712,-0.0651891902102615)) ;
#12100=DIRECTION('ref_axis',(0.924216281275222,0.380918326637037,-0.0269349931843281)) ;
#12101=DIRECTION('center_axis',(-0.381869435050519,-0.921914369154711,0.0651891902102615)) ;
#12102=DIRECTION('ref_axis',(0.92421628127522,-0.38091832663704,0.0269349931843284)) ;
#12103=DIRECTION('center_axis',(-0.381869435050519,-0.921914369154711,0.0651891902102615)) ;
#12104=DIRECTION('ref_axis',(0.92421628127522,-0.38091832663704,0.0269349931843284)) ;
#12105=DIRECTION('center_axis',(0.,0.,1.)) ;
#12106=DIRECTION('ref_axis',(-0.707106781186548,0.707106781186548,0.)) ;
#12107=DIRECTION('center_axis',(0.381869435050519,0.921914369154711,-0.0651891902102615)) ;
#12108=DIRECTION('ref_axis',(0.92421628127522,-0.38091832663704,0.0269349931843284)) ;
#12109=DIRECTION('center_axis',(0.381869435050519,0.921914369154711,-0.0651891902102615)) ;
#12110=DIRECTION('ref_axis',(0.92421628127522,-0.38091832663704,0.0269349931843284)) ;
#12111=DIRECTION('center_axis',(-0.921914369154711,-0.381869435050518,0.0651891902102602)) ;
#12112=DIRECTION('ref_axis',(0.387393722130433,-0.908767745068235,0.155136358012956)) ;
#12113=DIRECTION('center_axis',(-0.921914369154711,-0.381869435050518,0.0651891902102602)) ;
#12114=DIRECTION('ref_axis',(0.387393722130433,-0.908767745068235,0.155136358012956)) ;
#12115=DIRECTION('center_axis',(0.,0.,1.)) ;
#12116=DIRECTION('ref_axis',(1.,0.,0.)) ;
#12117=DIRECTION('center_axis',(0.921914369154711,0.381869435050518,-0.0651891902102602)) ;
#12118=DIRECTION('ref_axis',(0.387393722130433,-0.908767745068235,0.155136358012956)) ;
#12119=DIRECTION('center_axis',(0.921914369154711,0.381869435050518,-0.0651891902102602)) ;
#12120=DIRECTION('ref_axis',(0.387393722130433,-0.908767745068235,0.155136358012956)) ;
#12121=DIRECTION('center_axis',(-0.921914369154711,0.381869435050518,0.065189190210263)) ;
#12122=DIRECTION('ref_axis',(0.387393722130433,0.908767745068234,0.155136358012963)) ;
#12123=DIRECTION('center_axis',(0.,0.,1.)) ;
#12124=DIRECTION('ref_axis',(1.,0.,0.)) ;
#12125=DIRECTION('center_axis',(0.921914369154711,-0.381869435050518,-0.065189190210263)) ;
#12126=DIRECTION('ref_axis',(0.387393722130433,0.908767745068234,0.155136358012963)) ;
#12127=DIRECTION('center_axis',(-0.381869435050518,0.921914369154711,0.0651891902102615)) ;
#12128=DIRECTION('ref_axis',(0.924216281275221,0.380918326637039,0.0269349931843283)) ;
#12129=DIRECTION('center_axis',(0.,0.,1.)) ;
#12130=DIRECTION('ref_axis',(1.,0.,0.)) ;
#12131=DIRECTION('center_axis',(0.381869435050518,-0.921914369154711,-0.0651891902102615)) ;
#12132=DIRECTION('ref_axis',(0.924216281275221,0.380918326637039,0.0269349931843283)) ;
#12133=DIRECTION('center_axis',(0.381869435050518,0.921914369154711,0.0651891902102614)) ;
#12134=DIRECTION('ref_axis',(0.924216281275221,-0.38091832663704,-0.0269349931843283)) ;
#12135=DIRECTION('center_axis',(0.,0.,1.)) ;
#12136=DIRECTION('ref_axis',(1.,0.,0.)) ;
#12137=DIRECTION('center_axis',(-0.381869435050518,-0.921914369154711,-0.0651891902102614)) ;
#12138=DIRECTION('ref_axis',(0.924216281275221,-0.38091832663704,-0.0269349931843283)) ;
#12139=DIRECTION('center_axis',(0.921914369154711,0.381869435050518,0.0651891902102602)) ;
#12140=DIRECTION('ref_axis',(0.387393722130433,-0.908767745068235,-0.155136358012956)) ;
#12141=DIRECTION('center_axis',(0.,0.,1.)) ;
#12142=DIRECTION('ref_axis',(1.,0.,0.)) ;
#12143=DIRECTION('center_axis',(-0.921914369154711,-0.381869435050518,-0.0651891902102602)) ;
#12144=DIRECTION('ref_axis',(0.387393722130433,-0.908767745068235,-0.155136358012956)) ;
#12145=DIRECTION('center_axis',(0.921914369154711,-0.381869435050517,0.0651891902102614)) ;
#12146=DIRECTION('ref_axis',(0.387393722130433,0.908767745068235,-0.155136358012959)) ;
#12147=DIRECTION('center_axis',(0.921914369154711,-0.381869435050517,0.0651891902102614)) ;
#12148=DIRECTION('ref_axis',(0.387393722130433,0.908767745068235,-0.155136358012959)) ;
#12149=DIRECTION('center_axis',(0.,0.,1.)) ;
#12150=DIRECTION('ref_axis',(-0.707106781186586,-0.707106781186509,0.)) ;
#12151=DIRECTION('center_axis',(-0.921914369154711,0.381869435050517,-0.0651891902102614)) ;
#12152=DIRECTION('ref_axis',(0.387393722130433,0.908767745068235,-0.155136358012959)) ;
#12153=DIRECTION('center_axis',(-0.921914369154711,0.381869435050517,-0.0651891902102614)) ;
#12154=DIRECTION('ref_axis',(0.387393722130433,0.908767745068235,-0.155136358012959)) ;
#12155=DIRECTION('center_axis',(0.381869435050516,-0.921914369154712,0.0651891902102629)) ;
#12156=DIRECTION('ref_axis',(0.924216281275222,0.380918326637037,-0.0269349931843287)) ;
#12157=DIRECTION('center_axis',(0.381869435050516,-0.921914369154712,0.0651891902102629)) ;
#12158=DIRECTION('ref_axis',(0.924216281275222,0.380918326637037,-0.0269349931843287)) ;
#12159=DIRECTION('center_axis',(0.,0.,1.)) ;
#12160=DIRECTION('ref_axis',(-1.,-1.55431223447522E-13,0.)) ;
#12161=DIRECTION('center_axis',(-0.381869435050516,0.921914369154712,-0.0651891902102629)) ;
#12162=DIRECTION('ref_axis',(0.924216281275222,0.380918326637037,-0.0269349931843287)) ;
#12163=DIRECTION('center_axis',(-0.381869435050516,0.921914369154712,-0.0651891902102629)) ;
#12164=DIRECTION('ref_axis',(0.924216281275222,0.380918326637037,-0.0269349931843287)) ;
#12165=DIRECTION('center_axis',(-0.381869435050519,-0.921914369154711,0.0651891902102608)) ;
#12166=DIRECTION('ref_axis',(0.92421628127522,-0.38091832663704,0.0269349931843281)) ;
#12167=DIRECTION('center_axis',(-0.381869435050519,-0.921914369154711,0.0651891902102608)) ;
#12168=DIRECTION('ref_axis',(0.92421628127522,-0.38091832663704,0.0269349931843281)) ;
#12169=DIRECTION('center_axis',(0.,0.,1.)) ;
#12170=DIRECTION('ref_axis',(-0.70710678118647,0.707106781186625,0.)) ;
#12171=DIRECTION('center_axis',(0.381869435050519,0.921914369154711,-0.0651891902102608)) ;
#12172=DIRECTION('ref_axis',(0.92421628127522,-0.38091832663704,0.0269349931843281)) ;
#12173=DIRECTION('center_axis',(0.381869435050519,0.921914369154711,-0.0651891902102608)) ;
#12174=DIRECTION('ref_axis',(0.92421628127522,-0.38091832663704,0.0269349931843281)) ;
#12175=DIRECTION('center_axis',(-0.921914369154711,-0.381869435050518,0.0651891902102616)) ;
#12176=DIRECTION('ref_axis',(0.387393722130434,-0.908767745068234,0.155136358012959)) ;
#12177=DIRECTION('center_axis',(-0.921914369154711,-0.381869435050518,0.0651891902102616)) ;
#12178=DIRECTION('ref_axis',(0.387393722130434,-0.908767745068234,0.155136358012959)) ;
#12179=DIRECTION('center_axis',(0.,0.,1.)) ;
#12180=DIRECTION('ref_axis',(1.,0.,0.)) ;
#12181=DIRECTION('center_axis',(0.921914369154711,0.381869435050518,-0.0651891902102616)) ;
#12182=DIRECTION('ref_axis',(0.387393722130434,-0.908767745068234,0.155136358012959)) ;
#12183=DIRECTION('center_axis',(0.921914369154711,0.381869435050518,-0.0651891902102616)) ;
#12184=DIRECTION('ref_axis',(0.387393722130434,-0.908767745068234,0.155136358012959)) ;
#12185=DIRECTION('center_axis',(-0.921914369154711,0.381869435050518,0.0651891902102608)) ;
#12186=DIRECTION('ref_axis',(0.387393722130433,0.908767745068235,0.155136358012958)) ;
#12187=DIRECTION('center_axis',(0.,0.,1.)) ;
#12188=DIRECTION('ref_axis',(1.,0.,0.)) ;
#12189=DIRECTION('center_axis',(0.921914369154711,-0.381869435050518,-0.0651891902102608)) ;
#12190=DIRECTION('ref_axis',(0.387393722130433,0.908767745068235,0.155136358012958)) ;
#12191=DIRECTION('center_axis',(-0.381869435050518,0.921914369154711,0.0651891902102615)) ;
#12192=DIRECTION('ref_axis',(0.924216281275221,0.380918326637039,0.0269349931843283)) ;
#12193=DIRECTION('center_axis',(0.,0.,1.)) ;
#12194=DIRECTION('ref_axis',(1.,0.,0.)) ;
#12195=DIRECTION('center_axis',(0.381869435050518,-0.921914369154711,-0.0651891902102615)) ;
#12196=DIRECTION('ref_axis',(0.924216281275221,0.380918326637039,0.0269349931843283)) ;
#12197=DIRECTION('center_axis',(0.381869435050517,0.921914369154711,0.0651891902102621)) ;
#12198=DIRECTION('ref_axis',(0.924216281275221,-0.380918326637038,-0.0269349931843285)) ;
#12199=DIRECTION('center_axis',(0.,0.,1.)) ;
#12200=DIRECTION('ref_axis',(1.,0.,0.)) ;
#12201=DIRECTION('center_axis',(-0.381869435050517,-0.921914369154711,-0.0651891902102621)) ;
#12202=DIRECTION('ref_axis',(0.924216281275221,-0.380918326637038,-0.0269349931843285)) ;
#12203=DIRECTION('center_axis',(0.921914369154711,0.381869435050518,0.0651891902102615)) ;
#12204=DIRECTION('ref_axis',(0.387393722130433,-0.908767745068234,-0.155136358012959)) ;
#12205=DIRECTION('center_axis',(0.,0.,1.)) ;
#12206=DIRECTION('ref_axis',(1.,0.,0.)) ;
#12207=DIRECTION('center_axis',(-0.921914369154711,-0.381869435050518,-0.0651891902102615)) ;
#12208=DIRECTION('ref_axis',(0.387393722130433,-0.908767745068234,-0.155136358012959)) ;
#12209=DIRECTION('center_axis',(0.921914369154711,-0.381869435050517,0.0651891902102607)) ;
#12210=DIRECTION('ref_axis',(0.387393722130432,0.908767745068235,-0.155136358012958)) ;
#12211=DIRECTION('center_axis',(0.921914369154711,-0.381869435050517,0.0651891902102607)) ;
#12212=DIRECTION('ref_axis',(0.387393722130432,0.908767745068235,-0.155136358012958)) ;
#12213=DIRECTION('center_axis',(0.,0.,1.)) ;
#12214=DIRECTION('ref_axis',(-0.70710678118647,-0.707106781186625,0.)) ;
#12215=DIRECTION('center_axis',(-0.921914369154711,0.381869435050517,-0.0651891902102607)) ;
#12216=DIRECTION('ref_axis',(0.387393722130432,0.908767745068235,-0.155136358012958)) ;
#12217=DIRECTION('center_axis',(-0.921914369154711,0.381869435050517,-0.0651891902102607)) ;
#12218=DIRECTION('ref_axis',(0.387393722130432,0.908767745068235,-0.155136358012958)) ;
#12219=DIRECTION('center_axis',(0.381869435050516,-0.921914369154712,0.0651891902102615)) ;
#12220=DIRECTION('ref_axis',(0.924216281275222,0.380918326637037,-0.0269349931843281)) ;
#12221=DIRECTION('center_axis',(0.381869435050516,-0.921914369154712,0.0651891902102615)) ;
#12222=DIRECTION('ref_axis',(0.924216281275222,0.380918326637037,-0.0269349931843281)) ;
#12223=DIRECTION('center_axis',(0.,0.,1.)) ;
#12224=DIRECTION('ref_axis',(-1.,7.77156117237609E-14,0.)) ;
#12225=DIRECTION('center_axis',(-0.381869435050516,0.921914369154712,-0.0651891902102615)) ;
#12226=DIRECTION('ref_axis',(0.924216281275222,0.380918326637037,-0.0269349931843281)) ;
#12227=DIRECTION('center_axis',(-0.381869435050516,0.921914369154712,-0.0651891902102615)) ;
#12228=DIRECTION('ref_axis',(0.924216281275222,0.380918326637037,-0.0269349931843281)) ;
#12229=DIRECTION('center_axis',(-0.381869435050517,-0.921914369154712,0.0651891902102616)) ;
#12230=DIRECTION('ref_axis',(0.924216281275221,-0.380918326637038,0.0269349931843282)) ;
#12231=DIRECTION('center_axis',(-0.381869435050517,-0.921914369154712,0.0651891902102616)) ;
#12232=DIRECTION('ref_axis',(0.924216281275221,-0.380918326637038,0.0269349931843282)) ;
#12233=DIRECTION('center_axis',(0.,0.,1.)) ;
#12234=DIRECTION('ref_axis',(-0.707106781186431,0.707106781186664,0.)) ;
#12235=DIRECTION('center_axis',(0.381869435050517,0.921914369154712,-0.0651891902102616)) ;
#12236=DIRECTION('ref_axis',(0.924216281275221,-0.380918326637038,0.0269349931843282)) ;
#12237=DIRECTION('center_axis',(0.381869435050517,0.921914369154712,-0.0651891902102616)) ;
#12238=DIRECTION('ref_axis',(0.924216281275221,-0.380918326637038,0.0269349931843282)) ;
#12239=DIRECTION('center_axis',(-0.921914369154711,-0.381869435050517,0.0651891902102621)) ;
#12240=DIRECTION('ref_axis',(0.387393722130433,-0.908767745068234,0.155136358012961)) ;
#12241=DIRECTION('center_axis',(-0.921914369154711,-0.381869435050517,0.0651891902102621)) ;
#12242=DIRECTION('ref_axis',(0.387393722130433,-0.908767745068234,0.155136358012961)) ;
#12243=DIRECTION('center_axis',(0.,0.,1.)) ;
#12244=DIRECTION('ref_axis',(1.,0.,0.)) ;
#12245=DIRECTION('center_axis',(0.921914369154711,0.381869435050517,-0.0651891902102621)) ;
#12246=DIRECTION('ref_axis',(0.387393722130433,-0.908767745068234,0.155136358012961)) ;
#12247=DIRECTION('center_axis',(0.921914369154711,0.381869435050517,-0.0651891902102621)) ;
#12248=DIRECTION('ref_axis',(0.387393722130433,-0.908767745068234,0.155136358012961)) ;
#12249=DIRECTION('center_axis',(-0.921914369154711,0.381869435050518,0.0651891902102608)) ;
#12250=DIRECTION('ref_axis',(0.387393722130433,0.908767745068235,0.155136358012958)) ;
#12251=DIRECTION('center_axis',(0.,0.,1.)) ;
#12252=DIRECTION('ref_axis',(1.,0.,0.)) ;
#12253=DIRECTION('center_axis',(0.921914369154711,-0.381869435050518,-0.0651891902102608)) ;
#12254=DIRECTION('ref_axis',(0.387393722130433,0.908767745068235,0.155136358012958)) ;
#12255=DIRECTION('center_axis',(-0.381869435050518,0.921914369154711,0.0651891902102615)) ;
#12256=DIRECTION('ref_axis',(0.924216281275221,0.380918326637039,0.0269349931843283)) ;
#12257=DIRECTION('center_axis',(0.381869435050518,0.921914369154711,0.0651891902102614)) ;
#12258=DIRECTION('ref_axis',(0.924216281275221,-0.38091832663704,-0.0269349931843283)) ;
#12259=DIRECTION('center_axis',(0.381869435050518,0.921914369154711,0.0651891902102614)) ;
#12260=DIRECTION('ref_axis',(0.924216281275221,-0.38091832663704,-0.0269349931843283)) ;
#12261=DIRECTION('',(-0.381869435050518,-0.921914369154711,-0.0651891902102614)) ;
#12262=DIRECTION('center_axis',(-0.705345615858608,-0.705345615858589,-0.0705345615858606)) ;
#12263=DIRECTION('ref_axis',(0.707106781186538,-0.707106781186557,1.08220028400547E-15)) ;
#12264=DIRECTION('center_axis',(-0.705345615858608,-0.705345615858589,-0.0705345615858606)) ;
#12265=DIRECTION('ref_axis',(0.707106781186538,-0.707106781186557,1.08220028400547E-15)) ;
#12266=DIRECTION('center_axis',(-0.705345615858608,-0.705345615858589,-0.0705345615858606)) ;
#12267=DIRECTION('ref_axis',(0.707106781186538,-0.707106781186557,1.08220028400547E-15)) ;
#12268=DIRECTION('center_axis',(0.381869435050518,0.921914369154711,0.0651891902102614)) ;
#12269=DIRECTION('ref_axis',(0.924216281275221,-0.38091832663704,-0.0269349931843283)) ;
#12270=DIRECTION('center_axis',(0.921914369154713,0.381869435050514,0.0651891902102614)) ;
#12271=DIRECTION('ref_axis',(0.38739372213043,-0.908767745068236,-0.155136358012961)) ;
#12272=DIRECTION('',(-0.921914369154712,-0.381869435050514,-0.0651891902102614)) ;
#12273=DIRECTION('center_axis',(-0.997509336107633,-7.23745399280958E-16,
-0.0705345615858551)) ;
#12274=DIRECTION('ref_axis',(1.43792352550728E-15,-1.,-1.06215953800537E-14)) ;
#12275=DIRECTION('center_axis',(-0.997509336107633,-7.23745399280958E-16,
-0.0705345615858551)) ;
#12276=DIRECTION('ref_axis',(1.43792352550728E-15,-1.,-1.06215953800537E-14)) ;
#12277=DIRECTION('center_axis',(0.921914369154711,-0.381869435050519,0.0651891902102617)) ;
#12278=DIRECTION('ref_axis',(0.387393722130434,0.908767745068234,-0.155136358012959)) ;
#12279=DIRECTION('',(-0.921914369154711,0.381869435050519,-0.0651891902102617)) ;
#12280=DIRECTION('center_axis',(-0.705345615858604,0.705345615858592,-0.0705345615858606)) ;
#12281=DIRECTION('ref_axis',(0.707106781186541,0.707106781186554,-1.54313744200781E-15)) ;
#12282=DIRECTION('center_axis',(0.381869435050516,-0.921914369154712,0.0651891902102615)) ;
#12283=DIRECTION('ref_axis',(0.924216281275222,0.380918326637037,-0.0269349931843281)) ;
#12284=DIRECTION('',(-0.381869435050516,0.921914369154712,-0.0651891902102615)) ;
#12285=DIRECTION('center_axis',(0.,0.997509336107633,-0.0705345615858551)) ;
#12286=DIRECTION('ref_axis',(1.,0.,0.)) ;
#12287=DIRECTION('center_axis',(-0.381869435050518,-0.921914369154711,0.0651891902102613)) ;
#12288=DIRECTION('ref_axis',(0.924216281275221,-0.380918326637039,0.0269349931843282)) ;
#12289=DIRECTION('',(0.381869435050518,0.921914369154711,-0.0651891902102613)) ;
#12290=DIRECTION('center_axis',(0.705345615858603,0.705345615858593,-0.0705345615858606)) ;
#12291=DIRECTION('ref_axis',(0.707106781186542,-0.707106781186553,-1.76358564800892E-15)) ;
#12292=DIRECTION('center_axis',(-0.921914369154711,-0.381869435050517,0.0651891902102618)) ;
#12293=DIRECTION('ref_axis',(0.387393722130432,-0.908767745068235,0.15513635801296)) ;
#12294=DIRECTION('',(0.921914369154711,0.381869435050517,-0.0651891902102618)) ;
#12295=DIRECTION('center_axis',(0.997509336107633,-1.02353055936833E-14,
-0.0705345615858551)) ;
#12296=DIRECTION('ref_axis',(-9.27636030479688E-15,-1.,1.27859959480646E-14)) ;
#12297=DIRECTION('center_axis',(0.997509336107633,-1.02353055936833E-14,
-0.0705345615858551)) ;
#12298=DIRECTION('ref_axis',(-9.27636030479688E-15,-1.,1.27859959480646E-14)) ;
#12299=DIRECTION('center_axis',(-0.921914369154711,0.381869435050517,0.0651891902102614)) ;
#12300=DIRECTION('ref_axis',(0.387393722130432,0.908767745068235,0.155136358012959)) ;
#12301=DIRECTION('',(0.921914369154711,-0.381869435050517,-0.0651891902102613)) ;
#12302=DIRECTION('center_axis',(0.705345615858604,-0.705345615858593,-0.0705345615858606)) ;
#12303=DIRECTION('ref_axis',(0.707106781186542,0.707106781186553,2.56521548801298E-15)) ;
#12304=DIRECTION('center_axis',(0.705345615858604,-0.705345615858593,-0.0705345615858606)) ;
#12305=DIRECTION('ref_axis',(0.707106781186542,0.707106781186553,2.56521548801298E-15)) ;
#12306=DIRECTION('center_axis',(0.705345615858604,-0.705345615858593,-0.0705345615858606)) ;
#12307=DIRECTION('ref_axis',(0.707106781186542,0.707106781186553,2.56521548801298E-15)) ;
#12308=DIRECTION('center_axis',(-0.381869435050518,0.921914369154711,0.0651891902102615)) ;
#12309=DIRECTION('ref_axis',(0.924216281275221,0.380918326637039,0.0269349931843283)) ;
#12310=DIRECTION('',(0.381869435050518,-0.921914369154711,-0.0651891902102615)) ;
#12311=DIRECTION('center_axis',(-1.02353055936834E-14,-0.997509336107633,
-0.0705345615858551)) ;
#12312=DIRECTION('ref_axis',(1.,-1.01806989680515E-14,-7.16456669503621E-16)) ;
#12313=DIRECTION('center_axis',(-1.02353055936834E-14,-0.997509336107633,
-0.0705345615858551)) ;
#12314=DIRECTION('ref_axis',(1.,-1.01806989680515E-14,-7.16456669503621E-16)) ;
#12315=DIRECTION('center_axis',(0.381869435050518,0.921914369154711,0.0651891902102614)) ;
#12316=DIRECTION('ref_axis',(0.924216281275221,-0.38091832663704,-0.0269349931843283)) ;
#12317=DIRECTION('',(-0.381869435050518,-0.921914369154711,-0.0651891902102614)) ;
#12318=DIRECTION('center_axis',(-0.705345615858608,-0.705345615858589,-0.0705345615858606)) ;
#12319=DIRECTION('ref_axis',(0.707106781186538,-0.707106781186557,1.08220028400547E-15)) ;
#12320=DIRECTION('center_axis',(-0.705345615858608,-0.705345615858589,-0.0705345615858606)) ;
#12321=DIRECTION('ref_axis',(0.707106781186538,-0.707106781186557,1.08220028400547E-15)) ;
#12322=DIRECTION('center_axis',(-0.705345615858608,-0.705345615858589,-0.0705345615858606)) ;
#12323=DIRECTION('ref_axis',(0.707106781186538,-0.707106781186557,1.08220028400547E-15)) ;
#12324=DIRECTION('center_axis',(0.921914369154711,0.381869435050517,0.0651891902102614)) ;
#12325=DIRECTION('ref_axis',(0.387393722130433,-0.908767745068235,-0.155136358012959)) ;
#12326=DIRECTION('',(-0.921914369154711,-0.381869435050517,-0.0651891902102614)) ;
#12327=DIRECTION('center_axis',(-0.997509336107633,-1.44749079856192E-15,
-0.0705345615858551)) ;
#12328=DIRECTION('ref_axis',(2.24706864526137E-15,-1.,-1.05815138880535E-14)) ;
#12329=DIRECTION('center_axis',(-0.997509336107633,-1.44749079856192E-15,
-0.0705345615858551)) ;
#12330=DIRECTION('ref_axis',(2.24706864526137E-15,-1.,-1.05815138880535E-14)) ;
#12331=DIRECTION('center_axis',(0.921914369154711,-0.381869435050518,0.0651891902102616)) ;
#12332=DIRECTION('ref_axis',(0.387393722130434,0.908767745068234,-0.155136358012959)) ;
#12333=DIRECTION('',(-0.921914369154711,0.381869435050518,-0.0651891902102616)) ;
#12334=DIRECTION('center_axis',(-0.705345615858604,0.705345615858592,-0.0705345615858606)) ;
#12335=DIRECTION('ref_axis',(0.707106781186541,0.707106781186554,-1.60325968000812E-15)) ;
#12336=DIRECTION('center_axis',(0.381869435050516,-0.921914369154712,0.0651891902102615)) ;
#12337=DIRECTION('ref_axis',(0.924216281275222,0.380918326637037,-0.0269349931843281)) ;
#12338=DIRECTION('',(-0.381869435050516,0.921914369154712,-0.0651891902102615)) ;
#12339=DIRECTION('center_axis',(1.02353055936834E-14,0.997509336107633,
-0.0705345615858551)) ;
#12340=DIRECTION('ref_axis',(1.,-1.02207804600517E-14,7.21466856003647E-16)) ;
#12341=DIRECTION('center_axis',(-0.381869435050519,-0.921914369154711,0.0651891902102615)) ;
#12342=DIRECTION('ref_axis',(0.92421628127522,-0.38091832663704,0.0269349931843284)) ;
#12343=DIRECTION('',(0.381869435050519,0.92191436915471,-0.0651891902102615)) ;
#12344=DIRECTION('center_axis',(0.705345615858598,0.705345615858598,-0.0705345615858606)) ;
#12345=DIRECTION('ref_axis',(0.707106781186547,-0.707106781186548,-1.79364676700907E-15)) ;
#12346=DIRECTION('center_axis',(-0.921914369154711,-0.381869435050518,0.0651891902102602)) ;
#12347=DIRECTION('ref_axis',(0.387393722130433,-0.908767745068235,0.155136358012956)) ;
#12348=DIRECTION('',(0.921914369154711,0.381869435050518,-0.0651891902102602)) ;
#12349=DIRECTION('center_axis',(0.997509336107633,-1.09590509929644E-14,
-0.0705345615858551)) ;
#12350=DIRECTION('ref_axis',(-1.03861166145525E-14,-1.,8.47723555804284E-15)) ;
#12351=DIRECTION('center_axis',(0.997509336107633,-1.09590509929644E-14,
-0.0705345615858551)) ;
#12352=DIRECTION('ref_axis',(-1.03861166145525E-14,-1.,8.47723555804284E-15)) ;
#12353=DIRECTION('center_axis',(-0.921914369154711,0.381869435050518,0.065189190210263)) ;
#12354=DIRECTION('ref_axis',(0.387393722130433,0.908767745068234,0.155136358012963)) ;
#12355=DIRECTION('',(0.921914369154711,-0.381869435050518,-0.065189190210263)) ;
#12356=DIRECTION('center_axis',(0.705345615858598,-0.705345615858599,-0.0705345615858606)) ;
#12357=DIRECTION('ref_axis',(0.707106781186548,0.707106781186547,-2.20448206001115E-15)) ;
#12358=DIRECTION('center_axis',(0.705345615858598,-0.705345615858599,-0.0705345615858606)) ;
#12359=DIRECTION('ref_axis',(0.707106781186548,0.707106781186547,-2.20448206001115E-15)) ;
#12360=DIRECTION('center_axis',(0.705345615858598,-0.705345615858599,-0.0705345615858606)) ;
#12361=DIRECTION('ref_axis',(0.707106781186548,0.707106781186547,-2.20448206001115E-15)) ;
#12362=DIRECTION('center_axis',(-0.381869435050518,0.921914369154711,0.0651891902102615)) ;
#12363=DIRECTION('ref_axis',(0.924216281275221,0.380918326637039,0.0269349931843283)) ;
#12364=DIRECTION('',(0.381869435050518,-0.921914369154711,-0.0651891902102615)) ;
#12365=DIRECTION('center_axis',(-1.02353055936834E-14,-0.997509336107633,
-0.0705345615858551)) ;
#12366=DIRECTION('ref_axis',(1.,-1.01806989680515E-14,-7.16456669503621E-16)) ;
#12367=DIRECTION('center_axis',(-1.02353055936834E-14,-0.997509336107633,
-0.0705345615858551)) ;
#12368=DIRECTION('ref_axis',(1.,-1.01806989680515E-14,-7.16456669503621E-16)) ;
#12369=DIRECTION('center_axis',(0.381869435050518,0.921914369154711,0.0651891902102614)) ;
#12370=DIRECTION('ref_axis',(0.924216281275221,-0.38091832663704,-0.0269349931843283)) ;
#12371=DIRECTION('',(-0.381869435050518,-0.921914369154711,-0.0651891902102614)) ;
#12372=DIRECTION('center_axis',(-0.705345615858604,-0.705345615858593,-0.0705345615858606)) ;
#12373=DIRECTION('ref_axis',(0.707106781186542,-0.707106781186553,1.5631781880079E-15)) ;
#12374=DIRECTION('center_axis',(-0.705345615858604,-0.705345615858593,-0.0705345615858606)) ;
#12375=DIRECTION('ref_axis',(0.707106781186542,-0.707106781186553,1.5631781880079E-15)) ;
#12376=DIRECTION('center_axis',(-0.705345615858604,-0.705345615858593,-0.0705345615858606)) ;
#12377=DIRECTION('ref_axis',(0.707106781186542,-0.707106781186553,1.5631781880079E-15)) ;
#12378=DIRECTION('center_axis',(0.921914369154711,0.381869435050518,0.0651891902102602)) ;
#12379=DIRECTION('ref_axis',(0.387393722130433,-0.908767745068235,-0.155136358012956)) ;
#12380=DIRECTION('',(-0.921914369154711,-0.381869435050518,-0.0651891902102602)) ;
#12381=DIRECTION('center_axis',(-0.997509336107633,1.02353055936834E-14,
-0.0705345615858551)) ;
#12382=DIRECTION('ref_axis',(-9.60953770704856E-15,-1.,-8.47723555804284E-15)) ;
#12383=DIRECTION('center_axis',(-0.997509336107633,1.02353055936834E-14,
-0.0705345615858551)) ;
#12384=DIRECTION('ref_axis',(-9.60953770704856E-15,-1.,-8.47723555804284E-15)) ;
#12385=DIRECTION('center_axis',(0.921914369154711,-0.381869435050517,0.0651891902102614)) ;
#12386=DIRECTION('ref_axis',(0.387393722130433,0.908767745068235,-0.155136358012959)) ;
#12387=DIRECTION('',(-0.921914369154711,0.381869435050517,-0.0651891902102614)) ;
#12388=DIRECTION('center_axis',(-0.705345615858599,0.705345615858598,-0.070534561585861)) ;
#12389=DIRECTION('ref_axis',(0.707106781186547,0.707106781186548,-2.50509325001267E-15)) ;
#12390=DIRECTION('center_axis',(0.381869435050516,-0.921914369154712,0.0651891902102629)) ;
#12391=DIRECTION('ref_axis',(0.924216281275222,0.380918326637037,-0.0269349931843287)) ;
#12392=DIRECTION('',(-0.381869435050516,0.921914369154712,-0.0651891902102629)) ;
#12393=DIRECTION('center_axis',(1.02353055936834E-14,0.997509336107633,
-0.0705345615858553)) ;
#12394=DIRECTION('ref_axis',(1.,-1.02207804600517E-14,7.31487229003697E-16)) ;
#12395=DIRECTION('center_axis',(-0.381869435050519,-0.921914369154711,0.0651891902102608)) ;
#12396=DIRECTION('ref_axis',(0.92421628127522,-0.38091832663704,0.0269349931843281)) ;
#12397=DIRECTION('',(0.381869435050519,0.92191436915471,-0.0651891902102608)) ;
#12398=DIRECTION('center_axis',(0.705345615858598,0.705345615858598,-0.0705345615858606)) ;
#12399=DIRECTION('ref_axis',(0.707106781186547,-0.707106781186548,-3.78770099401916E-15)) ;
#12400=DIRECTION('center_axis',(-0.921914369154711,-0.381869435050518,0.0651891902102616)) ;
#12401=DIRECTION('ref_axis',(0.387393722130434,-0.908767745068234,0.155136358012959)) ;
#12402=DIRECTION('',(0.921914369154711,0.381869435050518,-0.0651891902102616)) ;
#12403=DIRECTION('center_axis',(0.997509336107633,-7.2374539928096E-16,
-0.0705345615858553)) ;
#12404=DIRECTION('ref_axis',(1.42790315250722E-16,-1.,1.09422473160553E-14)) ;
#12405=DIRECTION('center_axis',(0.997509336107633,-7.2374539928096E-16,
-0.0705345615858553)) ;
#12406=DIRECTION('ref_axis',(1.42790315250722E-16,-1.,1.09422473160553E-14)) ;
#12407=DIRECTION('center_axis',(-0.921914369154711,0.381869435050518,0.0651891902102608)) ;
#12408=DIRECTION('ref_axis',(0.387393722130433,0.908767745068235,0.155136358012958)) ;
#12409=DIRECTION('',(0.921914369154711,-0.381869435050518,-0.0651891902102608)) ;
#12410=DIRECTION('center_axis',(0.705345615858603,-0.705345615858593,-0.070534561585861)) ;
#12411=DIRECTION('ref_axis',(0.707106781186543,0.707106781186552,4.90998277002485E-15)) ;
#12412=DIRECTION('center_axis',(0.705345615858603,-0.705345615858593,-0.070534561585861)) ;
#12413=DIRECTION('ref_axis',(0.707106781186543,0.707106781186552,4.90998277002485E-15)) ;
#12414=DIRECTION('center_axis',(0.705345615858603,-0.705345615858593,-0.070534561585861)) ;
#12415=DIRECTION('ref_axis',(0.707106781186543,0.707106781186552,4.90998277002485E-15)) ;
#12416=DIRECTION('center_axis',(-0.381869435050518,0.921914369154711,0.0651891902102615)) ;
#12417=DIRECTION('ref_axis',(0.924216281275221,0.380918326637039,0.0269349931843283)) ;
#12418=DIRECTION('',(0.381869435050518,-0.921914369154711,-0.0651891902102615)) ;
#12419=DIRECTION('center_axis',(0.,-0.997509336107633,-0.0705345615858555)) ;
#12420=DIRECTION('ref_axis',(1.,4.00814920002027E-17,5.01018650002534E-18)) ;
#12421=DIRECTION('center_axis',(0.,-0.997509336107633,-0.0705345615858555)) ;
#12422=DIRECTION('ref_axis',(1.,4.00814920002027E-17,5.01018650002534E-18)) ;
#12423=DIRECTION('center_axis',(0.381869435050517,0.921914369154711,0.0651891902102621)) ;
#12424=DIRECTION('ref_axis',(0.924216281275221,-0.380918326637038,-0.0269349931843285)) ;
#12425=DIRECTION('',(-0.381869435050517,-0.921914369154711,-0.0651891902102621)) ;
#12426=DIRECTION('center_axis',(-0.705345615858593,-0.705345615858604,-0.070534561585861)) ;
#12427=DIRECTION('ref_axis',(0.707106781186553,-0.707106781186542,1.43291333900725E-15)) ;
#12428=DIRECTION('center_axis',(-0.705345615858593,-0.705345615858604,-0.070534561585861)) ;
#12429=DIRECTION('ref_axis',(0.707106781186553,-0.707106781186542,1.43291333900725E-15)) ;
#12430=DIRECTION('center_axis',(-0.705345615858593,-0.705345615858604,-0.070534561585861)) ;
#12431=DIRECTION('ref_axis',(0.707106781186553,-0.707106781186542,1.43291333900725E-15)) ;
#12432=DIRECTION('center_axis',(0.921914369154711,0.381869435050518,0.0651891902102615)) ;
#12433=DIRECTION('ref_axis',(0.387393722130433,-0.908767745068234,-0.155136358012959)) ;
#12434=DIRECTION('',(-0.921914369154711,-0.381869435050518,-0.0651891902102615)) ;
#12435=DIRECTION('center_axis',(-0.997509336107633,3.61872699640481E-16,
-0.0705345615858555)) ;
#12436=DIRECTION('ref_axis',(4.65947344502357E-16,-1.,-1.07217991100542E-14)) ;
#12437=DIRECTION('center_axis',(-0.997509336107633,3.61872699640481E-16,
-0.0705345615858555)) ;
#12438=DIRECTION('ref_axis',(4.65947344502357E-16,-1.,-1.07217991100542E-14)) ;
#12439=DIRECTION('center_axis',(0.921914369154711,-0.381869435050517,0.0651891902102607)) ;
#12440=DIRECTION('ref_axis',(0.387393722130432,0.908767745068235,-0.155136358012958)) ;
#12441=DIRECTION('',(-0.921914369154711,0.381869435050517,-0.0651891902102607)) ;
#12442=DIRECTION('center_axis',(-0.705345615858603,0.705345615858593,-0.070534561585861)) ;
#12443=DIRECTION('ref_axis',(0.707106781186543,0.707106781186552,-5.17051246802617E-15)) ;
#12444=DIRECTION('center_axis',(0.381869435050516,-0.921914369154712,0.0651891902102615)) ;
#12445=DIRECTION('ref_axis',(0.924216281275222,0.380918326637037,-0.0269349931843281)) ;
#12446=DIRECTION('',(-0.381869435050516,0.921914369154712,-0.0651891902102615)) ;
#12447=DIRECTION('center_axis',(0.,0.997509336107633,-0.0705345615858555)) ;
#12448=DIRECTION('ref_axis',(1.,0.,0.)) ;
#12449=DIRECTION('center_axis',(-0.381869435050517,-0.921914369154712,0.0651891902102616)) ;
#12450=DIRECTION('ref_axis',(0.924216281275221,-0.380918326637038,0.0269349931843282)) ;
#12451=DIRECTION('',(0.381869435050517,0.921914369154711,-0.0651891902102615)) ;
#12452=DIRECTION('center_axis',(0.705345615858583,0.705345615858614,-0.070534561585861)) ;
#12453=DIRECTION('ref_axis',(0.707106781186563,-0.707106781186532,-4.02818994602041E-15)) ;
#12454=DIRECTION('center_axis',(-0.921914369154711,-0.381869435050517,0.0651891902102621)) ;
#12455=DIRECTION('ref_axis',(0.387393722130433,-0.908767745068234,0.155136358012961)) ;
#12456=DIRECTION('',(0.921914369154711,0.381869435050517,-0.0651891902102621)) ;
#12457=DIRECTION('center_axis',(0.997509336107633,-9.87343289404283E-15,
-0.0705345615858555)) ;
#12458=DIRECTION('ref_axis',(-8.91312178354505E-15,-1.,1.31667701220665E-14)) ;
#12459=DIRECTION('center_axis',(0.997509336107633,-9.87343289404283E-15,
-0.0705345615858555)) ;
#12460=DIRECTION('ref_axis',(-8.91312178354505E-15,-1.,1.31667701220665E-14)) ;
#12461=DIRECTION('center_axis',(-0.921914369154711,0.381869435050518,0.0651891902102608)) ;
#12462=DIRECTION('ref_axis',(0.387393722130433,0.908767745068235,0.155136358012958)) ;
#12463=DIRECTION('',(0.921914369154711,-0.381869435050518,-0.0651891902102608)) ;
#12464=DIRECTION('center_axis',(0.705345615858603,-0.705345615858593,-0.070534561585861)) ;
#12465=DIRECTION('ref_axis',(0.707106781186543,0.707106781186552,4.90998277002485E-15)) ;
#12466=DIRECTION('center_axis',(0.705345615858603,-0.705345615858593,-0.070534561585861)) ;
#12467=DIRECTION('ref_axis',(0.707106781186543,0.707106781186552,4.90998277002485E-15)) ;
#12468=DIRECTION('center_axis',(0.705345615858603,-0.705345615858593,-0.070534561585861)) ;
#12469=DIRECTION('ref_axis',(0.707106781186543,0.707106781186552,4.90998277002485E-15)) ;
#12470=DIRECTION('center_axis',(-0.381869435050518,0.921914369154711,0.0651891902102615)) ;
#12471=DIRECTION('ref_axis',(0.924216281275221,0.380918326637039,0.0269349931843283)) ;
#12472=DIRECTION('',(0.381869435050518,-0.921914369154711,-0.0651891902102615)) ;
#12473=DIRECTION('center_axis',(0.381869435050518,-0.921914369154711,-0.0651891902102615)) ;
#12474=DIRECTION('ref_axis',(0.924216281275221,0.380918326637039,0.0269349931843283)) ;
#12475=DIRECTION('center_axis',(0.381869435050518,-0.921914369154711,-0.0651891902102615)) ;
#12476=DIRECTION('ref_axis',(-0.924216281275221,-0.380918326637039,-0.0269349931843283)) ;
#14684=CARTESIAN_POINT('',(0.,0.,0.)) ;
#14685=CARTESIAN_POINT('Origin',(-1.65857864376269,-1.89142135623731,1.19)) ;
#14686=CARTESIAN_POINT('',(-1.65758113442658,-1.8904238469012,1.17004981327785)) ;
#14687=CARTESIAN_POINT('',(-1.6595761530988,-1.89241886557342,1.20995018672215)) ;
#14688=CARTESIAN_POINT('Origin',(-1.65857864376269,-1.89142135623731,1.19)) ;
#14689=CARTESIAN_POINT('Origin',(-1.65857864376269,-1.89142135623731,1.19)) ;
#14690=CARTESIAN_POINT('Origin',(-1.8,-1.95,1.18)) ;
#14691=CARTESIAN_POINT('',(-1.79858930876828,-1.95,1.16004981327785)) ;
#14692=CARTESIAN_POINT('',(-1.80141069123172,-1.95,1.19995018672215)) ;
#14693=CARTESIAN_POINT('Origin',(-1.8,-1.95,1.18)) ;
#14694=CARTESIAN_POINT('',(-1.80774787444261,-1.96817535490137,1.18310272716026)) ;
#14695=CARTESIAN_POINT('Origin',(-1.8,-1.95,1.18)) ;
#14696=CARTESIAN_POINT('Origin',(-1.8,-1.95,1.18)) ;
#14697=CARTESIAN_POINT('Origin',(-1.94142135623731,-1.89142135623731,1.17)) ;
#14698=CARTESIAN_POINT('',(-1.9404238469012,-1.89241886557342,1.15004981327785)) ;
#14699=CARTESIAN_POINT('',(-1.94916923067992,-1.90959671113867,1.17310272716026)) ;
#14700=CARTESIAN_POINT('Origin',(-1.94142135623731,-1.89142135623731,1.17)) ;
#14701=CARTESIAN_POINT('',(-1.94241886557342,-1.8904238469012,1.18995018672215)) ;
#14702=CARTESIAN_POINT('Origin',(-1.94142135623731,-1.89142135623731,1.17)) ;
#14703=CARTESIAN_POINT('',(-1.95990568186281,-1.89903972277005,1.17053869986369)) ;
#14704=CARTESIAN_POINT('Origin',(-1.94142135623731,-1.89142135623731,1.17)) ;
#14705=CARTESIAN_POINT('Origin',(-1.94142135623731,-1.89142135623731,1.17)) ;
#14706=CARTESIAN_POINT('Origin',(-2.,-1.75,1.16)) ;
#14707=CARTESIAN_POINT('',(-2.,-1.75141069123172,1.14004981327785)) ;
#14708=CARTESIAN_POINT('',(-2.0184843256255,-1.75761836653274,1.16053869986369)) ;
#14709=CARTESIAN_POINT('Origin',(-2.,-1.75,1.16)) ;
#14710=CARTESIAN_POINT('',(-2.,-1.74858930876828,1.17995018672215)) ;
#14711=CARTESIAN_POINT('Origin',(-2.,-1.75,1.16)) ;
#14712=CARTESIAN_POINT('',(-2.0184843256255,-1.74238163346726,1.15946130013631)) ;
#14713=CARTESIAN_POINT('Origin',(-2.,-1.75,1.16)) ;
#14714=CARTESIAN_POINT('Origin',(-2.,-1.75,1.16)) ;
#14715=CARTESIAN_POINT('Origin',(-1.94142135623731,-1.60857864376269,1.15)) ;
#14716=CARTESIAN_POINT('',(-1.94241886557342,-1.6095761530988,1.13004981327785)) ;
#14717=CARTESIAN_POINT('',(-1.95990568186281,-1.60096027722995,1.14946130013631)) ;
#14718=CARTESIAN_POINT('Origin',(-1.94142135623731,-1.60857864376269,1.15)) ;
#14719=CARTESIAN_POINT('',(-1.9404238469012,-1.60758113442658,1.16995018672215)) ;
#14720=CARTESIAN_POINT('Origin',(-1.94142135623731,-1.60857864376269,1.15)) ;
#14721=CARTESIAN_POINT('',(-1.94916923067992,-1.59040328886133,1.14689727283974)) ;
#14722=CARTESIAN_POINT('Origin',(-1.94142135623731,-1.60857864376269,1.15)) ;
#14723=CARTESIAN_POINT('Origin',(-1.94142135623731,-1.60857864376269,1.15)) ;
#14724=CARTESIAN_POINT('Origin',(-1.8,-1.55,1.14)) ;
#14725=CARTESIAN_POINT('',(-1.80141069123172,-1.55,1.12004981327785)) ;
#14726=CARTESIAN_POINT('',(-1.80774787444261,-1.53182464509864,1.13689727283974)) ;
#14727=CARTESIAN_POINT('Origin',(-1.8,-1.55,1.14)) ;
#14728=CARTESIAN_POINT('',(-1.79858930876828,-1.55,1.15995018672215)) ;
#14729=CARTESIAN_POINT('Origin',(-1.8,-1.55,1.14)) ;
#14730=CARTESIAN_POINT('Origin',(-1.8,-1.55,1.14)) ;
#14731=CARTESIAN_POINT('Origin',(-1.65857864376269,-1.60857864376269,1.13)) ;
#14732=CARTESIAN_POINT('',(-1.6595761530988,-1.60758113442658,1.11004981327785)) ;
#14733=CARTESIAN_POINT('',(-1.65758113442658,-1.6095761530988,1.14995018672215)) ;
#14734=CARTESIAN_POINT('Origin',(-1.65857864376269,-1.60857864376269,1.13)) ;
#14735=CARTESIAN_POINT('Origin',(-1.65857864376269,-1.60857864376269,1.13)) ;
#14736=CARTESIAN_POINT('Origin',(-1.6,-1.75,1.12)) ;
#14737=CARTESIAN_POINT('',(-1.6,-1.74858930876828,1.10004981327785)) ;
#14738=CARTESIAN_POINT('',(-1.6,-1.75141069123172,1.13995018672215)) ;
#14739=CARTESIAN_POINT('Origin',(-1.6,-1.75,1.12)) ;
#14740=CARTESIAN_POINT('Origin',(-1.6,-1.75,1.12)) ;
#14741=CARTESIAN_POINT('Origin',(-1.65857864376269,-1.89142135623731,1.11)) ;
#14742=CARTESIAN_POINT('',(-1.65758113442658,-1.8904238469012,1.09004981327785)) ;
#14743=CARTESIAN_POINT('',(-1.6595761530988,-1.89241886557342,1.12995018672215)) ;
#14744=CARTESIAN_POINT('Origin',(-1.65857864376269,-1.89142135623731,1.11)) ;
#14745=CARTESIAN_POINT('Origin',(-1.65857864376269,-1.89142135623731,1.11)) ;
#14746=CARTESIAN_POINT('Origin',(-1.8,-1.95,1.1)) ;
#14747=CARTESIAN_POINT('',(-1.79858930876828,-1.95,1.08004981327785)) ;
#14748=CARTESIAN_POINT('',(-1.80141069123172,-1.95,1.11995018672215)) ;
#14749=CARTESIAN_POINT('Origin',(-1.8,-1.95,1.1)) ;
#14750=CARTESIAN_POINT('',(-1.80774787444261,-1.96817535490137,1.10310272716026)) ;
#14751=CARTESIAN_POINT('Origin',(-1.8,-1.95,1.1)) ;
#14752=CARTESIAN_POINT('Origin',(-1.8,-1.95,1.1)) ;
#14753=CARTESIAN_POINT('Origin',(-1.94142135623731,-1.89142135623731,1.09)) ;
#14754=CARTESIAN_POINT('',(-1.9404238469012,-1.89241886557342,1.07004981327785)) ;
#14755=CARTESIAN_POINT('',(-1.94916923067992,-1.90959671113867,1.09310272716026)) ;
#14756=CARTESIAN_POINT('Origin',(-1.94142135623731,-1.89142135623731,1.09)) ;
#14757=CARTESIAN_POINT('',(-1.94241886557342,-1.8904238469012,1.10995018672215)) ;
#14758=CARTESIAN_POINT('Origin',(-1.94142135623731,-1.89142135623731,1.09)) ;
#14759=CARTESIAN_POINT('',(-1.95990568186281,-1.89903972277005,1.09053869986369)) ;
#14760=CARTESIAN_POINT('Origin',(-1.94142135623731,-1.89142135623731,1.09)) ;
#14761=CARTESIAN_POINT('Origin',(-1.94142135623731,-1.89142135623731,1.09)) ;
#14762=CARTESIAN_POINT('Origin',(-2.,-1.75,1.08)) ;
#14763=CARTESIAN_POINT('',(-2.,-1.75141069123172,1.06004981327785)) ;
#14764=CARTESIAN_POINT('',(-2.0184843256255,-1.75761836653274,1.08053869986369)) ;
#14765=CARTESIAN_POINT('Origin',(-2.,-1.75,1.08)) ;
#14766=CARTESIAN_POINT('',(-2.,-1.74858930876828,1.09995018672215)) ;
#14767=CARTESIAN_POINT('Origin',(-2.,-1.75,1.08)) ;
#14768=CARTESIAN_POINT('',(-2.0184843256255,-1.74238163346726,1.07946130013631)) ;
#14769=CARTESIAN_POINT('Origin',(-2.,-1.75,1.08)) ;
#14770=CARTESIAN_POINT('Origin',(-2.,-1.75,1.08)) ;
#14771=CARTESIAN_POINT('Origin',(-1.94142135623731,-1.60857864376269,1.07)) ;
#14772=CARTESIAN_POINT('',(-1.94241886557342,-1.6095761530988,1.05004981327785)) ;
#14773=CARTESIAN_POINT('',(-1.95990568186281,-1.60096027722995,1.06946130013631)) ;
#14774=CARTESIAN_POINT('Origin',(-1.94142135623731,-1.60857864376269,1.07)) ;
#14775=CARTESIAN_POINT('',(-1.9404238469012,-1.60758113442658,1.08995018672215)) ;
#14776=CARTESIAN_POINT('Origin',(-1.94142135623731,-1.60857864376269,1.07)) ;
#14777=CARTESIAN_POINT('',(-1.94916923067992,-1.59040328886133,1.06689727283974)) ;
#14778=CARTESIAN_POINT('Origin',(-1.94142135623731,-1.60857864376269,1.07)) ;
#14779=CARTESIAN_POINT('Origin',(-1.94142135623731,-1.60857864376269,1.07)) ;
#14780=CARTESIAN_POINT('Origin',(-1.8,-1.55,1.06)) ;
#14781=CARTESIAN_POINT('',(-1.80141069123172,-1.55,1.04004981327785)) ;
#14782=CARTESIAN_POINT('',(-1.80774787444261,-1.53182464509864,1.05689727283974)) ;
#14783=CARTESIAN_POINT('Origin',(-1.8,-1.55,1.06)) ;
#14784=CARTESIAN_POINT('',(-1.79858930876828,-1.55,1.07995018672215)) ;
#14785=CARTESIAN_POINT('Origin',(-1.8,-1.55,1.06)) ;
#14786=CARTESIAN_POINT('Origin',(-1.8,-1.55,1.06)) ;
#14787=CARTESIAN_POINT('Origin',(-1.65857864376269,-1.60857864376269,1.05)) ;
#14788=CARTESIAN_POINT('',(-1.6595761530988,-1.60758113442658,1.03004981327785)) ;
#14789=CARTESIAN_POINT('',(-1.65758113442658,-1.6095761530988,1.06995018672215)) ;
#14790=CARTESIAN_POINT('Origin',(-1.65857864376269,-1.60857864376269,1.05)) ;
#14791=CARTESIAN_POINT('Origin',(-1.65857864376269,-1.60857864376269,1.05)) ;
#14792=CARTESIAN_POINT('Origin',(-1.6,-1.75,1.04)) ;
#14793=CARTESIAN_POINT('',(-1.6,-1.74858930876828,1.02004981327785)) ;
#14794=CARTESIAN_POINT('',(-1.6,-1.75141069123172,1.05995018672215)) ;
#14795=CARTESIAN_POINT('Origin',(-1.6,-1.75,1.04)) ;
#14796=CARTESIAN_POINT('Origin',(-1.6,-1.75,1.04)) ;
#14797=CARTESIAN_POINT('Origin',(-1.65857864376269,-1.89142135623731,1.03)) ;
#14798=CARTESIAN_POINT('',(-1.65758113442658,-1.8904238469012,1.01004981327785)) ;
#14799=CARTESIAN_POINT('',(-1.6595761530988,-1.89241886557342,1.04995018672215)) ;
#14800=CARTESIAN_POINT('Origin',(-1.65857864376269,-1.89142135623731,1.03)) ;
#14801=CARTESIAN_POINT('Origin',(-1.65857864376269,-1.89142135623731,1.03)) ;
#14802=CARTESIAN_POINT('Origin',(-1.8,-1.95,1.02)) ;
#14803=CARTESIAN_POINT('',(-1.79858930876828,-1.95,1.00004981327785)) ;
#14804=CARTESIAN_POINT('',(-1.80141069123172,-1.95,1.03995018672215)) ;
#14805=CARTESIAN_POINT('Origin',(-1.8,-1.95,1.02)) ;
#14806=CARTESIAN_POINT('',(-1.80774787444261,-1.96817535490136,1.02310272716026)) ;
#14807=CARTESIAN_POINT('Origin',(-1.8,-1.95,1.02)) ;
#14808=CARTESIAN_POINT('Origin',(-1.8,-1.95,1.02)) ;
#14809=CARTESIAN_POINT('Origin',(-1.94142135623731,-1.89142135623731,1.01)) ;
#14810=CARTESIAN_POINT('',(-1.9404238469012,-1.89241886557342,0.990049813277847)) ;
#14811=CARTESIAN_POINT('',(-1.94916923067992,-1.90959671113867,1.01310272716026)) ;
#14812=CARTESIAN_POINT('Origin',(-1.94142135623731,-1.89142135623731,1.01)) ;
#14813=CARTESIAN_POINT('',(-1.94241886557342,-1.8904238469012,1.02995018672215)) ;
#14814=CARTESIAN_POINT('Origin',(-1.94142135623731,-1.89142135623731,1.01)) ;
#14815=CARTESIAN_POINT('',(-1.95990568186281,-1.89903972277005,1.01053869986369)) ;
#14816=CARTESIAN_POINT('Origin',(-1.94142135623731,-1.89142135623731,1.01)) ;
#14817=CARTESIAN_POINT('Origin',(-1.94142135623731,-1.89142135623731,1.01)) ;
#14818=CARTESIAN_POINT('Origin',(-2.,-1.75,1.)) ;
#14819=CARTESIAN_POINT('',(-2.,-1.75141069123172,0.980049813277847)) ;
#14820=CARTESIAN_POINT('',(-2.0184843256255,-1.75761836653274,1.00053869986369)) ;
#14821=CARTESIAN_POINT('Origin',(-2.,-1.75,1.)) ;
#14822=CARTESIAN_POINT('',(-2.,-1.74858930876828,1.01995018672215)) ;
#14823=CARTESIAN_POINT('Origin',(-2.,-1.75,1.)) ;
#14824=CARTESIAN_POINT('',(-2.0184843256255,-1.74238163346726,0.999461300136314)) ;
#14825=CARTESIAN_POINT('Origin',(-2.,-1.75,1.)) ;
#14826=CARTESIAN_POINT('Origin',(-2.,-1.75,1.)) ;
#14827=CARTESIAN_POINT('Origin',(-1.94142135623731,-1.60857864376269,0.99)) ;
#14828=CARTESIAN_POINT('',(-1.94241886557342,-1.6095761530988,0.970049813277847)) ;
#14829=CARTESIAN_POINT('',(-1.95990568186281,-1.60096027722995,0.989461300136314)) ;
#14830=CARTESIAN_POINT('Origin',(-1.94142135623731,-1.60857864376269,0.99)) ;
#14831=CARTESIAN_POINT('',(-1.9404238469012,-1.60758113442658,1.00995018672215)) ;
#14832=CARTESIAN_POINT('Origin',(-1.94142135623731,-1.60857864376269,0.99)) ;
#14833=CARTESIAN_POINT('',(-1.94916923067992,-1.59040328886133,0.986897272839741)) ;
#14834=CARTESIAN_POINT('Origin',(-1.94142135623731,-1.60857864376269,0.99)) ;
#14835=CARTESIAN_POINT('Origin',(-1.94142135623731,-1.60857864376269,0.99)) ;
#14836=CARTESIAN_POINT('Origin',(-1.8,-1.55,0.98)) ;
#14837=CARTESIAN_POINT('',(-1.80141069123172,-1.55,0.960049813277847)) ;
#14838=CARTESIAN_POINT('',(-1.80774787444261,-1.53182464509864,0.976897272839741)) ;
#14839=CARTESIAN_POINT('Origin',(-1.8,-1.55,0.98)) ;
#14840=CARTESIAN_POINT('',(-1.79858930876828,-1.55,0.999950186722153)) ;
#14841=CARTESIAN_POINT('Origin',(-1.8,-1.55,0.98)) ;
#14842=CARTESIAN_POINT('Origin',(-1.8,-1.55,0.98)) ;
#14843=CARTESIAN_POINT('Origin',(-1.65857864376269,-1.60857864376269,0.97)) ;
#14844=CARTESIAN_POINT('',(-1.6595761530988,-1.60758113442658,0.950049813277848)) ;
#14845=CARTESIAN_POINT('',(-1.65758113442658,-1.6095761530988,0.989950186722153)) ;
#14846=CARTESIAN_POINT('Origin',(-1.65857864376269,-1.60857864376269,0.97)) ;
#14847=CARTESIAN_POINT('Origin',(-1.65857864376269,-1.60857864376269,0.97)) ;
#14848=CARTESIAN_POINT('Origin',(-1.6,-1.75,0.96)) ;
#14849=CARTESIAN_POINT('',(-1.6,-1.74858930876828,0.940049813277848)) ;
#14850=CARTESIAN_POINT('',(-1.6,-1.75141069123172,0.979950186722153)) ;
#14851=CARTESIAN_POINT('Origin',(-1.6,-1.75,0.96)) ;
#14852=CARTESIAN_POINT('Origin',(-1.6,-1.75,0.96)) ;
#14853=CARTESIAN_POINT('Origin',(-1.65857864376269,-1.89142135623731,0.95)) ;
#14854=CARTESIAN_POINT('',(-1.65758113442658,-1.8904238469012,0.930049813277848)) ;
#14855=CARTESIAN_POINT('',(-1.6595761530988,-1.89241886557342,0.969950186722153)) ;
#14856=CARTESIAN_POINT('Origin',(-1.65857864376269,-1.89142135623731,0.95)) ;
#14857=CARTESIAN_POINT('Origin',(-1.65857864376269,-1.89142135623731,0.95)) ;
#14858=CARTESIAN_POINT('Origin',(-1.8,-1.95,0.94)) ;
#14859=CARTESIAN_POINT('',(-1.79858930876828,-1.95,0.920049813277847)) ;
#14860=CARTESIAN_POINT('',(-1.80141069123172,-1.95,0.959950186722153)) ;
#14861=CARTESIAN_POINT('Origin',(-1.8,-1.95,0.94)) ;
#14862=CARTESIAN_POINT('',(-1.80774787444261,-1.96817535490136,0.943102727160259)) ;
#14863=CARTESIAN_POINT('Origin',(-1.8,-1.95,0.94)) ;
#14864=CARTESIAN_POINT('Origin',(-1.8,-1.95,0.94)) ;
#14865=CARTESIAN_POINT('Origin',(-1.94142135623731,-1.89142135623731,0.93)) ;
#14866=CARTESIAN_POINT('',(-1.9404238469012,-1.89241886557342,0.910049813277847)) ;
#14867=CARTESIAN_POINT('',(-1.94916923067992,-1.90959671113867,0.933102727160259)) ;
#14868=CARTESIAN_POINT('Origin',(-1.94142135623731,-1.89142135623731,0.93)) ;
#14869=CARTESIAN_POINT('',(-1.94241886557342,-1.8904238469012,0.949950186722153)) ;
#14870=CARTESIAN_POINT('Origin',(-1.94142135623731,-1.89142135623731,0.93)) ;
#14871=CARTESIAN_POINT('',(-1.95990568186281,-1.89903972277005,0.930538699863687)) ;
#14872=CARTESIAN_POINT('Origin',(-1.94142135623731,-1.89142135623731,0.93)) ;
#14873=CARTESIAN_POINT('Origin',(-1.94142135623731,-1.89142135623731,0.93)) ;
#14874=CARTESIAN_POINT('Origin',(-2.,-1.75,0.92)) ;
#14875=CARTESIAN_POINT('',(-2.,-1.75141069123172,0.900049813277847)) ;
#14876=CARTESIAN_POINT('',(-2.0184843256255,-1.75761836653274,0.920538699863687)) ;
#14877=CARTESIAN_POINT('Origin',(-2.,-1.75,0.92)) ;
#14878=CARTESIAN_POINT('',(-2.,-1.74858930876828,0.939950186722153)) ;
#14879=CARTESIAN_POINT('Origin',(-2.,-1.75,0.92)) ;
#14880=CARTESIAN_POINT('',(-2.0184843256255,-1.74238163346726,0.919461300136314)) ;
#14881=CARTESIAN_POINT('Origin',(-2.,-1.75,0.92)) ;
#14882=CARTESIAN_POINT('Origin',(-2.,-1.75,0.92)) ;
#14883=CARTESIAN_POINT('Origin',(-1.94142135623731,-1.60857864376269,0.91)) ;
#14884=CARTESIAN_POINT('',(-1.94241886557342,-1.6095761530988,0.890049813277848)) ;
#14885=CARTESIAN_POINT('',(-1.95990568186281,-1.60096027722995,0.909461300136314)) ;
#14886=CARTESIAN_POINT('Origin',(-1.94142135623731,-1.60857864376269,0.91)) ;
#14887=CARTESIAN_POINT('',(-1.9404238469012,-1.60758113442658,0.929950186722153)) ;
#14888=CARTESIAN_POINT('Origin',(-1.94142135623731,-1.60857864376269,0.91)) ;
#14889=CARTESIAN_POINT('',(-1.94916923067992,-1.59040328886133,0.906897272839741)) ;
#14890=CARTESIAN_POINT('Origin',(-1.94142135623731,-1.60857864376269,0.91)) ;
#14891=CARTESIAN_POINT('Origin',(-1.94142135623731,-1.60857864376269,0.91)) ;
#14892=CARTESIAN_POINT('Origin',(-1.8,-1.55,0.9)) ;
#14893=CARTESIAN_POINT('',(-1.80141069123172,-1.55,0.880049813277847)) ;
#14894=CARTESIAN_POINT('',(-1.80774787444261,-1.53182464509864,0.896897272839741)) ;
#14895=CARTESIAN_POINT('Origin',(-1.8,-1.55,0.9)) ;
#14896=CARTESIAN_POINT('',(-1.79858930876828,-1.55,0.919950186722153)) ;
#14897=CARTESIAN_POINT('Origin',(-1.8,-1.55,0.9)) ;
#14898=CARTESIAN_POINT('Origin',(-1.8,-1.55,0.9)) ;
#14899=CARTESIAN_POINT('Origin',(-1.65857864376269,-1.60857864376269,0.89)) ;
#14900=CARTESIAN_POINT('',(-1.6595761530988,-1.60758113442658,0.870049813277847)) ;
#14901=CARTESIAN_POINT('',(-1.65758113442658,-1.6095761530988,0.909950186722153)) ;
#14902=CARTESIAN_POINT('Origin',(-1.65857864376269,-1.60857864376269,0.89)) ;
#14903=CARTESIAN_POINT('Origin',(-1.65857864376269,-1.60857864376269,0.89)) ;
#14904=CARTESIAN_POINT('Origin',(-1.62928932188135,-1.82071067811866,1.195)) ;
#14905=CARTESIAN_POINT('',(-1.6184843256255,-1.74238163346726,1.20053869986369)) ;
#14906=CARTESIAN_POINT('Origin',(-1.6,-1.75,1.2)) ;
#14907=CARTESIAN_POINT('',(-1.67391193696982,-1.87619572450464,1.1910766147446)) ;
#14908=CARTESIAN_POINT('',(-1.64777364750685,-1.81309231158591,1.19553869986369)) ;
#14909=CARTESIAN_POINT('',(-1.67388148147355,-1.87637536958489,1.1925685105844)) ;
#14910=CARTESIAN_POINT('Origin',(-1.65857864376269,-1.89142135623731,1.19)) ;
#14911=CARTESIAN_POINT('Origin',(-1.65857864376269,-1.89142135623731,1.19)) ;
#14912=CARTESIAN_POINT('Origin',(-1.65857864376269,-1.89142135623731,1.19)) ;
#14913=CARTESIAN_POINT('Origin',(-1.6,-1.75,1.2)) ;
#14914=CARTESIAN_POINT('Origin',(-1.72928932188135,-1.92071067811866,1.185)) ;
#14915=CARTESIAN_POINT('',(-1.80025685105844,-1.92872176161686,1.18363242250356)) ;
#14916=CARTESIAN_POINT('',(-1.73703719632395,-1.90253532321729,1.18810272716026)) ;
#14917=CARTESIAN_POINT('Origin',(-1.8,-1.95,1.18)) ;
#14918=CARTESIAN_POINT('Origin',(-1.8,-1.95,1.18)) ;
#14919=CARTESIAN_POINT('Origin',(-1.87071067811866,-1.92071067811865,1.175)) ;
#14920=CARTESIAN_POINT('',(-1.87845855256126,-1.93888603302002,1.17810272716026)) ;
#14921=CARTESIAN_POINT('Origin',(-1.94142135623731,-1.89142135623731,1.17)) ;
#14922=CARTESIAN_POINT('Origin',(-1.97071067811865,-1.82071067811865,1.165)) ;
#14923=CARTESIAN_POINT('',(-1.98919500374416,-1.8283290446514,1.16553869986369)) ;
#14924=CARTESIAN_POINT('Origin',(-2.,-1.75,1.16)) ;
#14925=CARTESIAN_POINT('Origin',(-1.97071067811865,-1.67928932188134,1.155)) ;
#14926=CARTESIAN_POINT('',(-1.98919500374416,-1.6716709553486,1.15446130013631)) ;
#14927=CARTESIAN_POINT('Origin',(-1.94142135623731,-1.60857864376269,1.15)) ;
#14928=CARTESIAN_POINT('Origin',(-1.87071067811865,-1.57928932188135,1.145)) ;
#14929=CARTESIAN_POINT('',(-1.87845855256126,-1.56111396697998,1.14189727283974)) ;
#14930=CARTESIAN_POINT('',(-1.80025685105844,-1.57127823838314,1.13636757749644)) ;
#14931=CARTESIAN_POINT('Origin',(-1.8,-1.55,1.14)) ;
#14932=CARTESIAN_POINT('Origin',(-1.8,-1.55,1.14)) ;
#14933=CARTESIAN_POINT('Origin',(-1.72928932188135,-1.57928932188135,1.135)) ;
#14934=CARTESIAN_POINT('',(-1.67388148147355,-1.62362463041511,1.1274314894156)) ;
#14935=CARTESIAN_POINT('',(-1.73703719632395,-1.59746467678271,1.13189727283974)) ;
#14936=CARTESIAN_POINT('',(-1.67391193696982,-1.62380427549536,1.1289233852554)) ;
#14937=CARTESIAN_POINT('Origin',(-1.65857864376269,-1.60857864376269,1.13)) ;
#14938=CARTESIAN_POINT('Origin',(-1.65857864376269,-1.60857864376269,1.13)) ;
#14939=CARTESIAN_POINT('Origin',(-1.65857864376269,-1.60857864376269,1.13)) ;
#14940=CARTESIAN_POINT('Origin',(-1.62928932188135,-1.67928932188135,1.125)) ;
#14941=CARTESIAN_POINT('',(-1.6216399563665,-1.75,1.12)) ;
#14942=CARTESIAN_POINT('',(-1.64777364750685,-1.68690768841409,1.12446130013631)) ;
#14943=CARTESIAN_POINT('Origin',(-1.6,-1.75,1.12)) ;
#14944=CARTESIAN_POINT('Origin',(-1.6,-1.75,1.12)) ;
#14945=CARTESIAN_POINT('Origin',(-1.62928932188135,-1.82071067811865,1.115)) ;
#14946=CARTESIAN_POINT('',(-1.67391193696982,-1.87619572450464,1.1110766147446)) ;
#14947=CARTESIAN_POINT('',(-1.64777364750685,-1.81309231158591,1.11553869986369)) ;
#14948=CARTESIAN_POINT('',(-1.67388148147355,-1.87637536958489,1.1125685105844)) ;
#14949=CARTESIAN_POINT('Origin',(-1.65857864376269,-1.89142135623731,1.11)) ;
#14950=CARTESIAN_POINT('Origin',(-1.65857864376269,-1.89142135623731,1.11)) ;
#14951=CARTESIAN_POINT('Origin',(-1.65857864376269,-1.89142135623731,1.11)) ;
#14952=CARTESIAN_POINT('Origin',(-1.72928932188135,-1.92071067811865,1.105)) ;
#14953=CARTESIAN_POINT('',(-1.80025685105844,-1.92872176161686,1.10363242250356)) ;
#14954=CARTESIAN_POINT('',(-1.73703719632395,-1.90253532321729,1.10810272716026)) ;
#14955=CARTESIAN_POINT('Origin',(-1.8,-1.95,1.1)) ;
#14956=CARTESIAN_POINT('Origin',(-1.8,-1.95,1.1)) ;
#14957=CARTESIAN_POINT('Origin',(-1.87071067811866,-1.92071067811865,1.095)) ;
#14958=CARTESIAN_POINT('',(-1.87845855256126,-1.93888603302002,1.09810272716026)) ;
#14959=CARTESIAN_POINT('Origin',(-1.94142135623731,-1.89142135623731,1.09)) ;
#14960=CARTESIAN_POINT('Origin',(-1.97071067811865,-1.82071067811865,1.085)) ;
#14961=CARTESIAN_POINT('',(-1.98919500374416,-1.8283290446514,1.08553869986369)) ;
#14962=CARTESIAN_POINT('Origin',(-2.,-1.75,1.08)) ;
#14963=CARTESIAN_POINT('Origin',(-1.97071067811865,-1.67928932188135,1.075)) ;
#14964=CARTESIAN_POINT('',(-1.98919500374416,-1.6716709553486,1.07446130013631)) ;
#14965=CARTESIAN_POINT('Origin',(-1.94142135623731,-1.60857864376269,1.07)) ;
#14966=CARTESIAN_POINT('Origin',(-1.87071067811865,-1.57928932188135,1.065)) ;
#14967=CARTESIAN_POINT('',(-1.87845855256126,-1.56111396697998,1.06189727283974)) ;
#14968=CARTESIAN_POINT('',(-1.80025685105844,-1.57127823838314,1.05636757749644)) ;
#14969=CARTESIAN_POINT('Origin',(-1.8,-1.55,1.06)) ;
#14970=CARTESIAN_POINT('Origin',(-1.8,-1.55,1.06)) ;
#14971=CARTESIAN_POINT('Origin',(-1.72928932188135,-1.57928932188135,1.055)) ;
#14972=CARTESIAN_POINT('',(-1.67388148147355,-1.62362463041511,1.0474314894156)) ;
#14973=CARTESIAN_POINT('',(-1.73703719632395,-1.59746467678271,1.05189727283974)) ;
#14974=CARTESIAN_POINT('',(-1.67391193696982,-1.62380427549536,1.0489233852554)) ;
#14975=CARTESIAN_POINT('Origin',(-1.65857864376269,-1.60857864376269,1.05)) ;
#14976=CARTESIAN_POINT('Origin',(-1.65857864376269,-1.60857864376269,1.05)) ;
#14977=CARTESIAN_POINT('Origin',(-1.65857864376269,-1.60857864376269,1.05)) ;
#14978=CARTESIAN_POINT('Origin',(-1.62928932188135,-1.67928932188135,1.045)) ;
#14979=CARTESIAN_POINT('',(-1.6216399563665,-1.75,1.04)) ;
#14980=CARTESIAN_POINT('',(-1.64777364750685,-1.68690768841409,1.04446130013631)) ;
#14981=CARTESIAN_POINT('Origin',(-1.6,-1.75,1.04)) ;
#14982=CARTESIAN_POINT('Origin',(-1.6,-1.75,1.04)) ;
#14983=CARTESIAN_POINT('Origin',(-1.62928932188135,-1.82071067811865,1.035)) ;
#14984=CARTESIAN_POINT('',(-1.67391193696982,-1.87619572450464,1.0310766147446)) ;
#14985=CARTESIAN_POINT('',(-1.64777364750685,-1.81309231158591,1.03553869986369)) ;
#14986=CARTESIAN_POINT('',(-1.67388148147355,-1.87637536958489,1.0325685105844)) ;
#14987=CARTESIAN_POINT('Origin',(-1.65857864376269,-1.89142135623731,1.03)) ;
#14988=CARTESIAN_POINT('Origin',(-1.65857864376269,-1.89142135623731,1.03)) ;
#14989=CARTESIAN_POINT('Origin',(-1.65857864376269,-1.89142135623731,1.03)) ;
#14990=CARTESIAN_POINT('Origin',(-1.72928932188135,-1.92071067811865,1.025)) ;
#14991=CARTESIAN_POINT('',(-1.80025685105844,-1.92872176161686,1.02363242250356)) ;
#14992=CARTESIAN_POINT('',(-1.73703719632395,-1.90253532321729,1.02810272716026)) ;
#14993=CARTESIAN_POINT('Origin',(-1.8,-1.95,1.02)) ;
#14994=CARTESIAN_POINT('Origin',(-1.8,-1.95,1.02)) ;
#14995=CARTESIAN_POINT('Origin',(-1.87071067811865,-1.92071067811865,1.015)) ;
#14996=CARTESIAN_POINT('',(-1.87845855256126,-1.93888603302002,1.01810272716026)) ;
#14997=CARTESIAN_POINT('Origin',(-1.94142135623731,-1.89142135623731,1.01)) ;
#14998=CARTESIAN_POINT('Origin',(-1.97071067811865,-1.82071067811865,1.005)) ;
#14999=CARTESIAN_POINT('',(-1.98919500374416,-1.8283290446514,1.00553869986369)) ;
#15000=CARTESIAN_POINT('Origin',(-2.,-1.75,1.)) ;
#15001=CARTESIAN_POINT('Origin',(-1.97071067811865,-1.67928932188135,0.995)) ;
#15002=CARTESIAN_POINT('',(-1.98919500374416,-1.6716709553486,0.994461300136314)) ;
#15003=CARTESIAN_POINT('Origin',(-1.94142135623731,-1.60857864376269,0.99)) ;
#15004=CARTESIAN_POINT('Origin',(-1.87071067811865,-1.57928932188135,0.985)) ;
#15005=CARTESIAN_POINT('',(-1.87845855256126,-1.56111396697998,0.981897272839741)) ;
#15006=CARTESIAN_POINT('',(-1.80025685105844,-1.57127823838314,0.976367577496444)) ;
#15007=CARTESIAN_POINT('Origin',(-1.8,-1.55,0.98)) ;
#15008=CARTESIAN_POINT('Origin',(-1.8,-1.55,0.98)) ;
#15009=CARTESIAN_POINT('Origin',(-1.72928932188135,-1.57928932188135,0.975)) ;
#15010=CARTESIAN_POINT('',(-1.67388148147355,-1.62362463041511,0.967431489415601)) ;
#15011=CARTESIAN_POINT('',(-1.73703719632395,-1.59746467678271,0.971897272839741)) ;
#15012=CARTESIAN_POINT('',(-1.67391193696982,-1.62380427549536,0.968923385255398)) ;
#15013=CARTESIAN_POINT('Origin',(-1.65857864376269,-1.60857864376269,0.97)) ;
#15014=CARTESIAN_POINT('Origin',(-1.65857864376269,-1.60857864376269,0.97)) ;
#15015=CARTESIAN_POINT('Origin',(-1.65857864376269,-1.60857864376269,0.97)) ;
#15016=CARTESIAN_POINT('Origin',(-1.62928932188135,-1.67928932188135,0.965)) ;
#15017=CARTESIAN_POINT('',(-1.62163995636649,-1.75,0.96)) ;
#15018=CARTESIAN_POINT('',(-1.64777364750685,-1.68690768841409,0.964461300136314)) ;
#15019=CARTESIAN_POINT('Origin',(-1.6,-1.75,0.96)) ;
#15020=CARTESIAN_POINT('Origin',(-1.6,-1.75,0.96)) ;
#15021=CARTESIAN_POINT('Origin',(-1.62928932188135,-1.82071067811865,0.955)) ;
#15022=CARTESIAN_POINT('',(-1.67391193696982,-1.87619572450464,0.951076614744602)) ;
#15023=CARTESIAN_POINT('',(-1.64777364750685,-1.81309231158591,0.955538699863687)) ;
#15024=CARTESIAN_POINT('',(-1.67388148147355,-1.87637536958489,0.952568510584399)) ;
#15025=CARTESIAN_POINT('Origin',(-1.65857864376269,-1.89142135623731,0.95)) ;
#15026=CARTESIAN_POINT('Origin',(-1.65857864376269,-1.89142135623731,0.95)) ;
#15027=CARTESIAN_POINT('Origin',(-1.65857864376269,-1.89142135623731,0.95)) ;
#15028=CARTESIAN_POINT('Origin',(-1.72928932188135,-1.92071067811865,0.945)) ;
#15029=CARTESIAN_POINT('',(-1.80025685105844,-1.92872176161686,0.943632422503557)) ;
#15030=CARTESIAN_POINT('',(-1.73703719632395,-1.90253532321729,0.948102727160259)) ;
#15031=CARTESIAN_POINT('Origin',(-1.8,-1.95,0.94)) ;
#15032=CARTESIAN_POINT('Origin',(-1.8,-1.95,0.94)) ;
#15033=CARTESIAN_POINT('Origin',(-1.87071067811865,-1.92071067811865,0.935)) ;
#15034=CARTESIAN_POINT('',(-1.87845855256126,-1.93888603302002,0.938102727160259)) ;
#15035=CARTESIAN_POINT('Origin',(-1.94142135623731,-1.89142135623731,0.93)) ;
#15036=CARTESIAN_POINT('Origin',(-1.97071067811865,-1.82071067811865,0.925)) ;
#15037=CARTESIAN_POINT('',(-1.98919500374416,-1.8283290446514,0.925538699863687)) ;
#15038=CARTESIAN_POINT('Origin',(-2.,-1.75,0.92)) ;
#15039=CARTESIAN_POINT('Origin',(-1.97071067811865,-1.67928932188135,0.915)) ;
#15040=CARTESIAN_POINT('',(-1.98919500374416,-1.6716709553486,0.914461300136314)) ;
#15041=CARTESIAN_POINT('Origin',(-1.94142135623731,-1.60857864376269,0.91)) ;
#15042=CARTESIAN_POINT('Origin',(-1.87071067811865,-1.57928932188135,0.905)) ;
#15043=CARTESIAN_POINT('',(-1.87845855256126,-1.56111396697998,0.901897272839741)) ;
#15044=CARTESIAN_POINT('',(-1.80025685105844,-1.57127823838314,0.896367577496443)) ;
#15045=CARTESIAN_POINT('Origin',(-1.8,-1.55,0.9)) ;
#15046=CARTESIAN_POINT('Origin',(-1.8,-1.55,0.9)) ;
#15047=CARTESIAN_POINT('Origin',(-1.72928932188135,-1.57928932188135,0.895)) ;
#15048=CARTESIAN_POINT('',(-1.67388148147355,-1.62362463041511,0.887431489415601)) ;
#15049=CARTESIAN_POINT('',(-1.73703719632395,-1.59746467678271,0.891897272839741)) ;
#15050=CARTESIAN_POINT('',(-1.67391193696982,-1.62380427549536,0.888923385255398)) ;
#15051=CARTESIAN_POINT('Origin',(-1.65857864376269,-1.60857864376269,0.89)) ;
#15052=CARTESIAN_POINT('Origin',(-1.65857864376269,-1.60857864376269,0.89)) ;
#15053=CARTESIAN_POINT('Origin',(-1.65857864376269,-1.60857864376269,0.89)) ;
#15054=CARTESIAN_POINT('Origin',(-1.62928932188135,-1.67928932188135,0.885)) ;
#15055=CARTESIAN_POINT('',(-1.6184843256255,-1.75761836653274,0.879461300136314)) ;
#15056=CARTESIAN_POINT('',(-1.64777364750685,-1.68690768841409,0.884461300136314)) ;
#15057=CARTESIAN_POINT('Origin',(-1.6,-1.75,0.88)) ;
#15058=CARTESIAN_POINT('Origin',(-1.6,-1.75,0.88)) ;
#15429=UNCERTAINTY_MEASURE_WITH_UNIT(LENGTH_MEASURE(0.001),#15485,
'DISTANCE_ACCURACY_VALUE',
'Maximum model space distance between geometric entities at asserted c
onnectivities') ;
#15441=UNCERTAINTY_MEASURE_WITH_UNIT(LENGTH_MEASURE(0.001),#15485,
'DISTANCE_ACCURACY_VALUE',
'Maximum model space distance between geometric entities at asserted c
onnectivities') ;
#15472=(
GEOMETRIC_REPRESENTATION_CONTEXT(3)
GLOBAL_UNCERTAINTY_ASSIGNED_CONTEXT((#15429))
GLOBAL_UNIT_ASSIGNED_CONTEXT((#15485,#15487,#15488))
REPRESENTATION_CONTEXT('','3D')
) ;
#15484=(
GEOMETRIC_REPRESENTATION_CONTEXT(3)
GLOBAL_UNCERTAINTY_ASSIGNED_CONTEXT((#15441))
GLOBAL_UNIT_ASSIGNED_CONTEXT((#15485,#15487,#15488))
REPRESENTATION_CONTEXT('','3D')
) ;
#15485=(
LENGTH_UNIT()
NAMED_UNIT(*)
SI_UNIT(.CENTI.,.METRE.)
) ;
#15487=(
NAMED_UNIT(*)
PLANE_ANGLE_UNIT()
SI_UNIT($,.RADIAN.)
) ;
#15488=(
NAMED_UNIT(*)
SI_UNIT($,.STERADIAN.)
SOLID_ANGLE_UNIT()
) ;
#15519=SHAPE_DEFINITION_REPRESENTATION(#15576,#15648) ;
#15576=PRODUCT_DEFINITION_SHAPE('',$,#15691) ;
#15648=SHAPE_REPRESENTATION('',(#9548),#15472) ;
#15660=PRODUCT_DEFINITION_CONTEXT('part definition',#15788,'design') ;
#15691=PRODUCT_DEFINITION('CONTACT_PRESSURE_SPRING',
'CONTACT_PRESSURE_SPRING',#15733,#15660) ;
#15733=PRODUCT_DEFINITION_FORMATION('',$,#15820) ;
#15788=APPLICATION_CONTEXT(
'Core Data for Automotive Mechanical Design Process') ;
#15789=PRODUCT_CONTEXT('part definition',#15788,'mechanical') ;
#15820=PRODUCT('CONTACT_PRESSURE_SPRING','CONTACT_PRESSURE_SPRING',$,(#15789)) ;
#15832=PRESENTATION_STYLE_ASSIGNMENT((#15844)) ;
#15844=SURFACE_STYLE_USAGE(.BOTH.,#15856) ;
#15856=SURFACE_SIDE_STYLE('',(#15868)) ;
#15868=SURFACE_STYLE_FILL_AREA(#15880) ;
#15880=FILL_AREA_STYLE('Steel - Satin',(#15892)) ;
#15892=FILL_AREA_STYLE_COLOUR('Steel - Satin',#15904) ;
#15904=COLOUR_RGB('Steel - Satin', 0.72549020, 0.75294118, 0.79215686) ;
ENDSEC;
END-ISO-10303-21;
